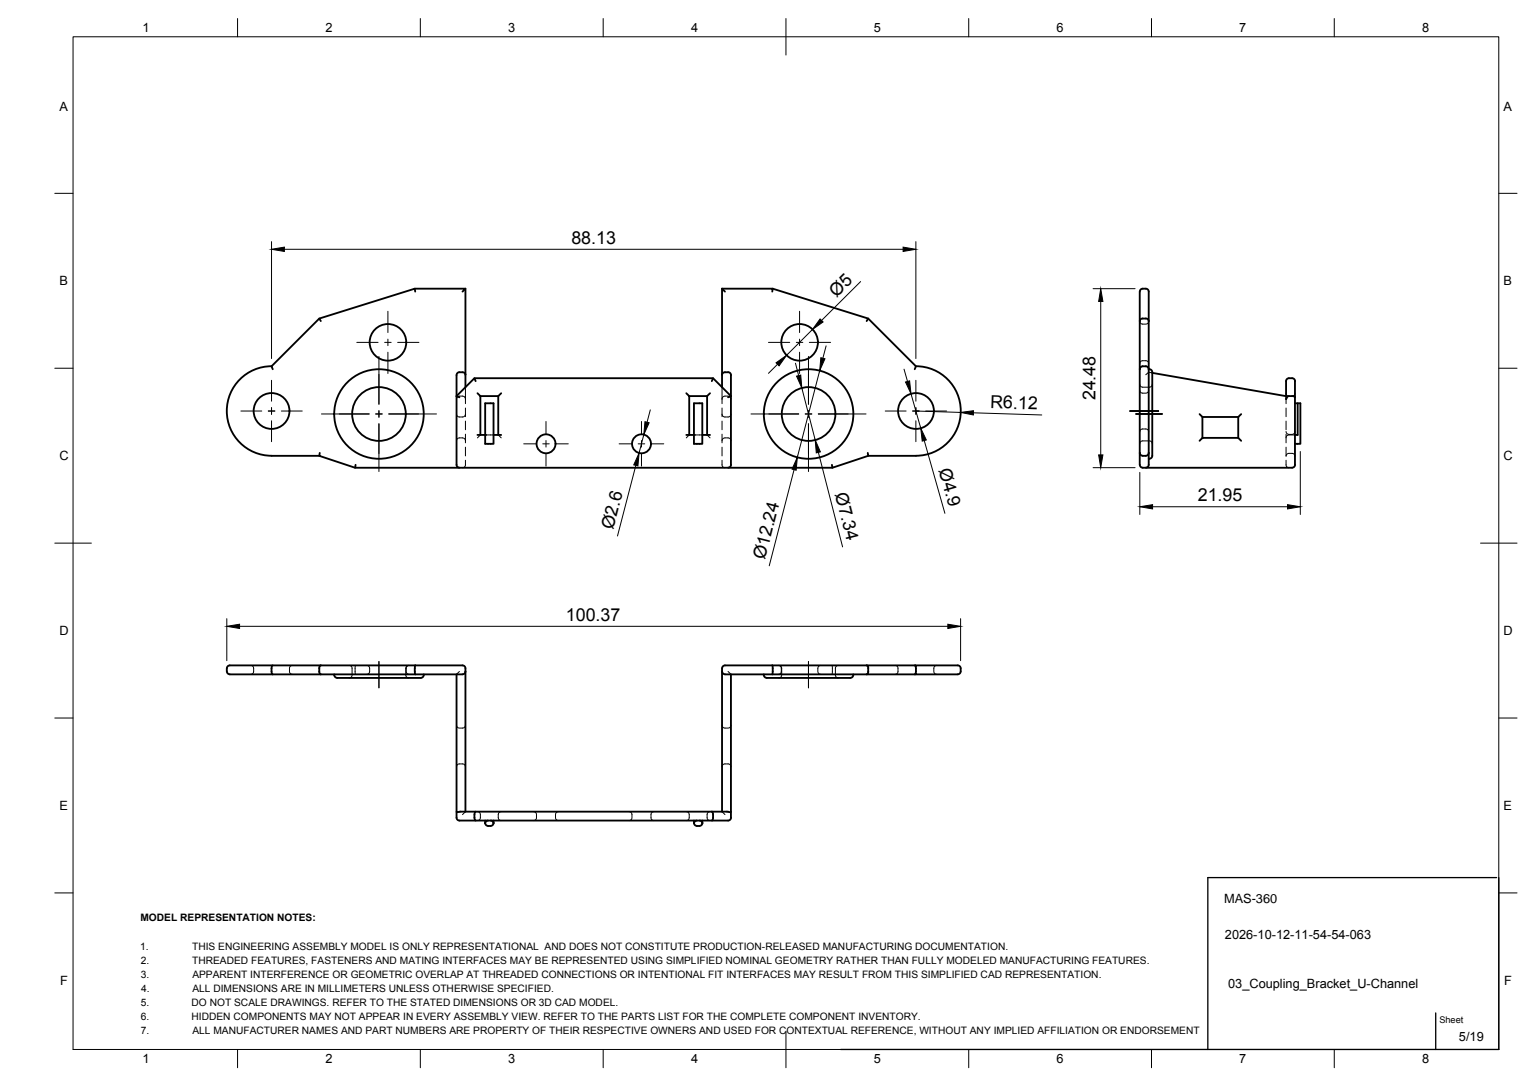
ISO-10303-21;
HEADER;
/* Generated by software containing ST-Developer
 * from STEP Tools, Inc. (www.steptools.com) 
 */

FILE_DESCRIPTION(
/* description */ (''),
/* implementation_level */ '2;1');

FILE_NAME(
/* name */ '03_Coupling_Bracket_U-Channel.step',
/* time_stamp */ '2026-11-04T18:53:29-08:00',
/* author */ (''),
/* organization */ (''),
/* preprocessor_version */ 'ST-DEVELOPER v20.2',
/* originating_system */ 'Autodesk Translation Framework v15.17.0.0',
/* authorisation */ '');

FILE_SCHEMA (('AUTOMOTIVE_DESIGN { 1 0 10303 214 3 1 1 }'));
ENDSEC;

DATA;
#10=MECHANICAL_DESIGN_GEOMETRIC_PRESENTATION_REPRESENTATION('',(#1329),#100031);
#181=SPHERICAL_SURFACE('',#20936,0.4);
#182=SPHERICAL_SURFACE('',#20950,0.4);
#183=SPHERICAL_SURFACE('',#20969,0.4);
#184=SPHERICAL_SURFACE('',#20993,0.4);
#540=CIRCLE('',#20937,0.4);
#541=CIRCLE('',#20938,0.4);
#542=CIRCLE('',#20939,0.399999999999999);
#543=CIRCLE('',#20951,0.400000000000003);
#544=CIRCLE('',#20952,0.399999999999999);
#545=CIRCLE('',#20953,0.400000000000001);
#546=CIRCLE('',#20965,0.4);
#547=CIRCLE('',#20970,0.4);
#548=CIRCLE('',#20971,0.400000000000001);
#549=CIRCLE('',#20972,0.399999999999999);
#550=CIRCLE('',#20977,5.72);
#551=CIRCLE('',#20978,6.12);
#552=CIRCLE('',#20984,6.12);
#553=CIRCLE('',#20992,0.4);
#554=CIRCLE('',#20994,0.399999999999999);
#555=CIRCLE('',#20995,0.4);
#556=CIRCLE('',#21012,0.4);
#557=CIRCLE('',#21014,6.12);
#558=CIRCLE('',#21015,5.72);
#559=CIRCLE('',#21025,6.12);
#560=CIRCLE('',#21032,0.400000000000009);
#561=CIRCLE('',#21033,5.72);
#562=CIRCLE('',#21041,4.072);
#563=CIRCLE('',#21042,2.848);
#564=CIRCLE('',#21043,2.9);
#565=CIRCLE('',#21045,5.72);
#566=CIRCLE('',#21046,0.4);
#567=CIRCLE('',#21047,6.12);
#568=CIRCLE('',#21048,6.12);
#569=CIRCLE('',#21050,4.072);
#570=CIRCLE('',#21052,6.12);
#571=CIRCLE('',#21054,0.4);
#572=CIRCLE('',#21065,5.72);
#573=CIRCLE('',#21067,4.072);
#574=CIRCLE('',#21068,2.9);
#575=CIRCLE('',#21069,2.848);
#576=CIRCLE('',#21071,5.72);
#577=CIRCLE('',#21072,0.4);
#578=CIRCLE('',#21073,6.12);
#579=CIRCLE('',#21074,6.12);
#580=CIRCLE('',#21076,4.072);
#581=CIRCLE('',#21078,6.12);
#582=CIRCLE('',#21080,0.4);
#583=CIRCLE('',#21081,3.672);
#584=CIRCLE('',#21082,3.672);
#585=CIRCLE('',#21084,3.672);
#586=CIRCLE('',#21085,3.672);
#587=CIRCLE('',#21087,0.4);
#588=CIRCLE('',#21089,0.4);
#589=CIRCLE('',#21090,3.672);
#590=CIRCLE('',#21091,3.672);
#591=CIRCLE('',#21093,3.672);
#592=CIRCLE('',#21094,3.672);
#593=CIRCLE('',#21096,0.4);
#594=CIRCLE('',#21098,0.4);
#595=CIRCLE('',#21099,2.448);
#596=CIRCLE('',#21100,2.448);
#597=CIRCLE('',#21102,2.448);
#598=CIRCLE('',#21103,2.448);
#599=CIRCLE('',#21105,2.848);
#600=CIRCLE('',#21106,0.4);
#601=CIRCLE('',#21108,2.9);
#602=CIRCLE('',#21110,0.4);
#603=CIRCLE('',#21111,2.5);
#604=CIRCLE('',#21112,2.5);
#605=CIRCLE('',#21114,2.5);
#606=CIRCLE('',#21115,2.5);
#607=CIRCLE('',#21117,2.9);
#608=CIRCLE('',#21118,0.4);
#609=CIRCLE('',#21120,2.848);
#610=CIRCLE('',#21122,0.4);
#611=CIRCLE('',#21123,2.5);
#612=CIRCLE('',#21124,2.5);
#613=CIRCLE('',#21126,2.5);
#614=CIRCLE('',#21127,2.5);
#615=CIRCLE('',#21129,0.4);
#616=CIRCLE('',#21131,0.4);
#617=CIRCLE('',#21132,2.448);
#618=CIRCLE('',#21133,2.448);
#619=CIRCLE('',#21135,2.448);
#620=CIRCLE('',#21136,2.448);
#621=CIRCLE('',#21138,0.4);
#622=CIRCLE('',#21140,1.7);
#623=CIRCLE('',#21141,0.4);
#624=CIRCLE('',#21142,1.3);
#625=CIRCLE('',#21143,1.3);
#626=CIRCLE('',#21145,1.3);
#627=CIRCLE('',#21146,1.3);
#628=CIRCLE('',#21148,1.7);
#629=CIRCLE('',#21160,1.7);
#630=CIRCLE('',#21161,0.4);
#631=CIRCLE('',#21163,1.7);
#632=CIRCLE('',#21172,0.4);
#633=CIRCLE('',#21173,1.3);
#634=CIRCLE('',#21174,1.3);
#635=CIRCLE('',#21176,1.3);
#636=CIRCLE('',#21177,1.3);
#637=CIRCLE('',#21179,0.4);
#638=CIRCLE('',#21191,0.4);
#639=CIRCLE('',#21196,0.4);
#640=CIRCLE('',#21209,0.4);
#641=CIRCLE('',#21214,0.4);
#642=CIRCLE('',#21217,0.4);
#643=CIRCLE('',#21218,0.4);
#644=CIRCLE('',#21219,0.4);
#645=CIRCLE('',#21221,0.4);
#646=CIRCLE('',#21222,0.4);
#647=CIRCLE('',#21224,0.4);
#648=CIRCLE('',#21225,0.4);
#649=CIRCLE('',#21228,0.4);
#650=CIRCLE('',#21229,0.4);
#651=CIRCLE('',#21231,0.4);
#652=CIRCLE('',#21237,0.4);
#653=CIRCLE('',#21238,0.4);
#654=CIRCLE('',#21239,0.4);
#655=CIRCLE('',#21241,0.4);
#656=CIRCLE('',#21242,0.4);
#657=CIRCLE('',#21244,0.4);
#658=CIRCLE('',#21245,0.4);
#659=CIRCLE('',#21248,0.4);
#660=CIRCLE('',#21249,0.4);
#661=CIRCLE('',#21251,0.4);
#1215=TOROIDAL_SURFACE('',#20976,5.72,0.4);
#1216=TOROIDAL_SURFACE('',#21013,5.72,0.4);
#1217=TOROIDAL_SURFACE('',#21031,5.72,0.4);
#1218=TOROIDAL_SURFACE('',#21044,5.72,0.4);
#1219=TOROIDAL_SURFACE('',#21064,5.72,0.4);
#1220=TOROIDAL_SURFACE('',#21070,5.72,0.4);
#1221=TOROIDAL_SURFACE('',#21079,4.072,0.4);
#1222=TOROIDAL_SURFACE('',#21086,4.072,0.4);
#1223=TOROIDAL_SURFACE('',#21088,4.072,0.4);
#1224=TOROIDAL_SURFACE('',#21095,4.072,0.4);
#1225=TOROIDAL_SURFACE('',#21097,2.848,0.4);
#1226=TOROIDAL_SURFACE('',#21104,2.848,0.4);
#1227=TOROIDAL_SURFACE('',#21109,2.9,0.4);
#1228=TOROIDAL_SURFACE('',#21116,2.9,0.4);
#1229=TOROIDAL_SURFACE('',#21121,2.9,0.4);
#1230=TOROIDAL_SURFACE('',#21128,2.9,0.4);
#1231=TOROIDAL_SURFACE('',#21130,2.848,0.4);
#1232=TOROIDAL_SURFACE('',#21137,2.848,0.4);
#1233=TOROIDAL_SURFACE('',#21139,1.7,0.4);
#1234=TOROIDAL_SURFACE('',#21159,1.7,0.4);
#1235=TOROIDAL_SURFACE('',#21171,1.7,0.4);
#1236=TOROIDAL_SURFACE('',#21178,1.7,0.4);
#1293=SHAPE_REPRESENTATION_RELATIONSHIP('SRR','None',#100103,#1311);
#1311=ADVANCED_BREP_SHAPE_REPRESENTATION('',(#1347),#100015);
#1329=STYLED_ITEM('',(#100201),#1347);
#1347=MANIFOLD_SOLID_BREP('Body1',#20119);
#1399=PLANE('',#20901);
#1400=PLANE('',#20902);
#1401=PLANE('',#20903);
#1402=PLANE('',#20915);
#1403=PLANE('',#20916);
#1404=PLANE('',#20922);
#1405=PLANE('',#20932);
#1406=PLANE('',#20933);
#1407=PLANE('',#20934);
#1408=PLANE('',#20942);
#1409=PLANE('',#20957);
#1410=PLANE('',#20980);
#1411=PLANE('',#20981);
#1412=PLANE('',#20982);
#1413=PLANE('',#20985);
#1414=PLANE('',#20986);
#1415=PLANE('',#21009);
#1416=PLANE('',#21010);
#1417=PLANE('',#21023);
#1418=PLANE('',#21026);
#1419=PLANE('',#21027);
#1420=PLANE('',#21028);
#1421=PLANE('',#21040);
#1422=PLANE('',#21049);
#1423=PLANE('',#21066);
#1424=PLANE('',#21075);
#1425=PLANE('',#21107);
#1426=PLANE('',#21119);
#1427=PLANE('',#21147);
#1428=PLANE('',#21155);
#1429=PLANE('',#21156);
#1430=PLANE('',#21157);
#1431=PLANE('',#21162);
#1432=PLANE('',#21188);
#1433=PLANE('',#21189);
#1434=PLANE('',#21197);
#1435=PLANE('',#21206);
#1436=PLANE('',#21207);
#1437=PLANE('',#21215);
#1438=PLANE('',#21223);
#1439=PLANE('',#21226);
#1440=PLANE('',#21227);
#1441=PLANE('',#21232);
#1442=PLANE('',#21233);
#1443=PLANE('',#21234);
#1444=PLANE('',#21243);
#1445=PLANE('',#21246);
#1446=PLANE('',#21247);
#1447=PLANE('',#21252);
#1448=PLANE('',#21253);
#1449=PLANE('',#21254);
#1450=PLANE('',#21256);
#1451=PLANE('',#21257);
#1452=PLANE('',#21258);
#1453=PLANE('',#21259);
#1454=PLANE('',#21260);
#1717=FACE_BOUND('',#6546,.T.);
#1718=FACE_BOUND('',#6554,.T.);
#1719=FACE_BOUND('',#6565,.T.);
#1720=FACE_BOUND('',#6604,.T.);
#1721=FACE_BOUND('',#6623,.T.);
#1722=FACE_BOUND('',#6624,.T.);
#1723=FACE_BOUND('',#6625,.T.);
#1724=FACE_BOUND('',#6628,.T.);
#1725=FACE_BOUND('',#6638,.T.);
#1726=FACE_BOUND('',#6639,.T.);
#1727=FACE_BOUND('',#6640,.T.);
#1728=FACE_BOUND('',#6643,.T.);
#1729=FACE_BOUND('',#6655,.T.);
#1730=FACE_BOUND('',#6656,.T.);
#1731=FACE_BOUND('',#6657,.T.);
#1732=FACE_BOUND('',#6662,.T.);
#1733=FACE_BOUND('',#6663,.T.);
#1734=FACE_BOUND('',#6664,.T.);
#1735=FACE_BOUND('',#6674,.T.);
#1736=FACE_BOUND('',#6675,.T.);
#1737=FACE_BOUND('',#6676,.T.);
#1738=FACE_BOUND('',#6677,.T.);
#1739=FACE_BOUND('',#6687,.T.);
#1740=FACE_BOUND('',#6688,.T.);
#1741=FACE_BOUND('',#6689,.T.);
#1742=FACE_BOUND('',#6690,.T.);
#1825=ELLIPSE('',#20894,0.565685424949238,0.4);
#1826=ELLIPSE('',#20895,0.565685424949238,0.4);
#1827=ELLIPSE('',#20897,0.565685424949238,0.4);
#1828=ELLIPSE('',#20899,0.565685424949238,0.4);
#1829=ELLIPSE('',#20904,0.565685424949239,0.4);
#1830=ELLIPSE('',#20906,0.406004087997522,0.4);
#1831=ELLIPSE('',#20908,0.565685424949238,0.4);
#1832=ELLIPSE('',#20909,0.565685424949238,0.4);
#1833=ELLIPSE('',#20911,0.565685424949238,0.4);
#1834=ELLIPSE('',#20912,0.565685424949238,0.4);
#1835=ELLIPSE('',#20918,0.522676873082012,0.4);
#1836=ELLIPSE('',#20919,0.406004087997522,0.4);
#1837=ELLIPSE('',#20921,0.406004087997522,0.4);
#1838=ELLIPSE('',#20923,0.574176487625014,0.4);
#1839=ELLIPSE('',#20925,0.565685424949238,0.4);
#1840=ELLIPSE('',#20926,0.565685424949238,0.4);
#1841=ELLIPSE('',#20928,0.565685424949238,0.4);
#1842=ELLIPSE('',#20930,0.565685424949238,0.4);
#1843=ELLIPSE('',#20935,0.565685424949239,0.4);
#1844=ELLIPSE('',#20941,0.565685424949238,0.4);
#1845=ELLIPSE('',#20944,0.405232582893276,0.4);
#1846=ELLIPSE('',#20946,0.565685424949238,0.4);
#1847=ELLIPSE('',#20948,0.56568542494924,0.4);
#1848=ELLIPSE('',#20949,0.405232582893277,0.4);
#1849=ELLIPSE('',#20956,0.405232582893276,0.4);
#1850=ELLIPSE('',#20959,0.565685424949238,0.4);
#1851=ELLIPSE('',#20961,0.404631208637699,0.4);
#1852=ELLIPSE('',#20963,0.41193011418047,0.4);
#1853=ELLIPSE('',#20966,0.405232582893276,0.4);
#1854=ELLIPSE('',#20968,0.405232582893276,0.4);
#1855=ELLIPSE('',#20974,0.565685424949237,0.4);
#1856=ELLIPSE('',#20989,0.43295688011696,0.4);
#1857=ELLIPSE('',#20991,0.565685424949238,0.4);
#1858=ELLIPSE('',#20997,0.405232582893276,0.4);
#1859=ELLIPSE('',#20999,0.522676873082012,0.4);
#1860=ELLIPSE('',#21000,0.406004087997522,0.4);
#1861=ELLIPSE('',#21002,0.565685424949238,0.4);
#1862=ELLIPSE('',#21003,0.565685424949238,0.4);
#1863=ELLIPSE('',#21005,0.565685424949238,0.4);
#1864=ELLIPSE('',#21006,0.565685424949238,0.4);
#1865=ELLIPSE('',#21017,0.41193011418047,0.4);
#1866=ELLIPSE('',#21019,0.404631208637698,0.4);
#1867=ELLIPSE('',#21021,0.56568542494924,0.4);
#1868=ELLIPSE('',#21030,0.405232582893276,0.4);
#1869=ELLIPSE('',#21036,0.411930114180469,0.4);
#1870=ELLIPSE('',#21038,0.404631208637699,0.4);
#1871=ELLIPSE('',#21055,0.405232582893276,0.4);
#1872=ELLIPSE('',#21058,0.565685424949238,0.4);
#1873=ELLIPSE('',#21060,0.404631208637698,0.4);
#1874=ELLIPSE('',#21062,0.411930114180471,0.4);
#1875=ELLIPSE('',#21150,0.574176487625014,0.4);
#1876=ELLIPSE('',#21151,0.432956880116957,0.4);
#1877=ELLIPSE('',#21153,0.432956880116958,0.4);
#1878=ELLIPSE('',#21165,0.432956880116959,0.4);
#1879=ELLIPSE('',#21166,0.432956880116958,0.4);
#1880=ELLIPSE('',#21169,0.432956880116958,0.4);
#1881=ELLIPSE('',#21181,0.565685424949238,0.4);
#1882=ELLIPSE('',#21182,0.565685424949238,0.4);
#1883=ELLIPSE('',#21184,0.565685424949238,0.4);
#1884=ELLIPSE('',#21186,0.565685424949238,0.4);
#1885=ELLIPSE('',#21192,0.565685424949238,0.4);
#1886=ELLIPSE('',#21194,0.565685424949238,0.4);
#1887=ELLIPSE('',#21199,0.565685424949238,0.4);
#1888=ELLIPSE('',#21200,0.565685424949238,0.4);
#1889=ELLIPSE('',#21202,0.565685424949238,0.4);
#1890=ELLIPSE('',#21204,0.565685424949238,0.4);
#1891=ELLIPSE('',#21210,0.565685424949238,0.4);
#1892=ELLIPSE('',#21212,0.565685424949238,0.4);
#2284=LINE('',#60104,#3571);
#2285=LINE('',#60108,#3572);
#2286=LINE('',#60112,#3573);
#2287=LINE('',#60114,#3574);
#2288=LINE('',#60118,#3575);
#2289=LINE('',#60120,#3576);
#2290=LINE('',#60123,#3577);
#2291=LINE('',#60124,#3578);
#2292=LINE('',#60127,#3579);
#2293=LINE('',#60129,#3580);
#2294=LINE('',#60130,#3581);
#2295=LINE('',#60133,#3582);
#2296=LINE('',#60134,#3583);
#2297=LINE('',#60138,#3584);
#2298=LINE('',#60142,#3585);
#2299=LINE('',#60144,#3586);
#2300=LINE('',#60146,#3587);
#2301=LINE('',#60147,#3588);
#2302=LINE('',#60168,#3589);
#2303=LINE('',#60172,#3590);
#2304=LINE('',#60175,#3591);
#2305=LINE('',#60180,#3592);
#2306=LINE('',#60184,#3593);
#2307=LINE('',#60186,#3594);
#2308=LINE('',#60187,#3595);
#2309=LINE('',#60189,#3596);
#2310=LINE('',#60193,#3597);
#2311=LINE('',#60195,#3598);
#2312=LINE('',#60197,#3599);
#2313=LINE('',#60199,#3600);
#2314=LINE('',#60201,#3601);
#2315=LINE('',#60202,#3602);
#2316=LINE('',#60208,#3603);
#2317=LINE('',#60229,#3604);
#2318=LINE('',#60232,#3605);
#2319=LINE('',#60237,#3606);
#2320=LINE('',#60239,#3607);
#2321=LINE('',#60240,#3608);
#2322=LINE('',#60244,#3609);
#2323=LINE('',#60248,#3610);
#2324=LINE('',#60252,#3611);
#2325=LINE('',#60254,#3612);
#2326=LINE('',#60258,#3613);
#2327=LINE('',#60260,#3614);
#2328=LINE('',#60263,#3615);
#2329=LINE('',#60264,#3616);
#2330=LINE('',#60267,#3617);
#2331=LINE('',#60269,#3618);
#2332=LINE('',#60270,#3619);
#2333=LINE('',#60273,#3620);
#2334=LINE('',#60274,#3621);
#2335=LINE('',#60277,#3622);
#2336=LINE('',#60279,#3623);
#2337=LINE('',#60281,#3624);
#2338=LINE('',#60283,#3625);
#2339=LINE('',#60294,#3626);
#2340=LINE('',#60297,#3627);
#2341=LINE('',#60299,#3628);
#2342=LINE('',#60301,#3629);
#2343=LINE('',#60303,#3630);
#2344=LINE('',#60305,#3631);
#2345=LINE('',#60307,#3632);
#2346=LINE('',#60309,#3633);
#2347=LINE('',#60311,#3634);
#2348=LINE('',#60313,#3635);
#2349=LINE('',#60315,#3636);
#2350=LINE('',#60316,#3637);
#2351=LINE('',#60319,#3638);
#2352=LINE('',#60324,#3639);
#2353=LINE('',#60328,#3640);
#2354=LINE('',#60338,#3641);
#2355=LINE('',#60341,#3642);
#2356=LINE('',#60344,#3643);
#2357=LINE('',#60345,#3644);
#2358=LINE('',#60348,#3645);
#2359=LINE('',#60352,#3646);
#2360=LINE('',#60355,#3647);
#2361=LINE('',#60358,#3648);
#2362=LINE('',#60361,#3649);
#2363=LINE('',#60365,#3650);
#2364=LINE('',#60369,#3651);
#2365=LINE('',#60373,#3652);
#2366=LINE('',#60375,#3653);
#2367=LINE('',#60384,#3654);
#2368=LINE('',#60419,#3655);
#2369=LINE('',#60420,#3656);
#2370=LINE('',#60423,#3657);
#2371=LINE('',#60424,#3658);
#2372=LINE('',#60427,#3659);
#2373=LINE('',#60428,#3660);
#2374=LINE('',#60431,#3661);
#2375=LINE('',#60432,#3662);
#2376=LINE('',#60435,#3663);
#2377=LINE('',#60439,#3664);
#2378=LINE('',#60440,#3665);
#2379=LINE('',#60442,#3666);
#2380=LINE('',#60444,#3667);
#2381=LINE('',#60448,#3668);
#2382=LINE('',#60454,#3669);
#2383=LINE('',#60462,#3670);
#2384=LINE('',#60468,#3671);
#2385=LINE('',#60472,#3672);
#2386=LINE('',#60475,#3673);
#2387=LINE('',#60480,#3674);
#2388=LINE('',#60484,#3675);
#2389=LINE('',#60486,#3676);
#2390=LINE('',#60487,#3677);
#2391=LINE('',#60489,#3678);
#2392=LINE('',#60492,#3679);
#2393=LINE('',#60494,#3680);
#2394=LINE('',#60495,#3681);
#2395=LINE('',#60496,#3682);
#2396=LINE('',#60501,#3683);
#2397=LINE('',#60502,#3684);
#2398=LINE('',#60538,#3685);
#2399=LINE('',#60541,#3686);
#2400=LINE('',#60544,#3687);
#2401=LINE('',#60547,#3688);
#2402=LINE('',#60550,#3689);
#2403=LINE('',#60553,#3690);
#2404=LINE('',#60554,#3691);
#2405=LINE('',#60557,#3692);
#2406=LINE('',#60558,#3693);
#2407=LINE('',#60561,#3694);
#2408=LINE('',#60565,#3695);
#2409=LINE('',#60566,#3696);
#2410=LINE('',#60569,#3697);
#2411=LINE('',#60570,#3698);
#2412=LINE('',#60572,#3699);
#2413=LINE('',#60575,#3700);
#2414=LINE('',#60611,#3701);
#2415=LINE('',#60614,#3702);
#2416=LINE('',#60618,#3703);
#2417=LINE('',#60621,#3704);
#2418=LINE('',#60642,#3705);
#2419=LINE('',#60648,#3706);
#2420=LINE('',#60651,#3707);
#2421=LINE('',#60654,#3708);
#2422=LINE('',#60658,#3709);
#2423=LINE('',#60662,#3710);
#2424=LINE('',#60666,#3711);
#2425=LINE('',#60717,#3712);
#2426=LINE('',#60727,#3713);
#2427=LINE('',#60741,#3714);
#2428=LINE('',#60758,#3715);
#2429=LINE('',#60777,#3716);
#2430=LINE('',#60783,#3717);
#2431=LINE('',#60797,#3718);
#2432=LINE('',#60811,#3719);
#2433=LINE('',#60827,#3720);
#2434=LINE('',#60831,#3721);
#2435=LINE('',#60832,#3722);
#2436=LINE('',#60833,#3723);
#2437=LINE('',#60835,#3724);
#2438=LINE('',#60836,#3725);
#2439=LINE('',#60841,#3726);
#2440=LINE('',#60843,#3727);
#2441=LINE('',#60845,#3728);
#2442=LINE('',#60846,#3729);
#2443=LINE('',#60849,#3730);
#2444=LINE('',#60851,#3731);
#2445=LINE('',#60853,#3732);
#2446=LINE('',#60854,#3733);
#2447=LINE('',#60857,#3734);
#2448=LINE('',#60863,#3735);
#2449=LINE('',#60865,#3736);
#2450=LINE('',#60868,#3737);
#2451=LINE('',#60869,#3738);
#2452=LINE('',#60872,#3739);
#2453=LINE('',#60873,#3740);
#2454=LINE('',#60875,#3741);
#2455=LINE('',#60883,#3742);
#2456=LINE('',#60885,#3743);
#2457=LINE('',#60887,#3744);
#2458=LINE('',#60888,#3745);
#2459=LINE('',#60891,#3746);
#2460=LINE('',#60893,#3747);
#2461=LINE('',#60895,#3748);
#2462=LINE('',#60897,#3749);
#2463=LINE('',#60899,#3750);
#2464=LINE('',#60901,#3751);
#2465=LINE('',#60903,#3752);
#2466=LINE('',#60904,#3753);
#2467=LINE('',#60907,#3754);
#2468=LINE('',#60909,#3755);
#2469=LINE('',#60911,#3756);
#2470=LINE('',#60913,#3757);
#2471=LINE('',#60915,#3758);
#2472=LINE('',#60917,#3759);
#2473=LINE('',#60919,#3760);
#2474=LINE('',#60920,#3761);
#2475=LINE('',#60938,#3762);
#2476=LINE('',#60948,#3763);
#2477=LINE('',#60952,#3764);
#2478=LINE('',#60956,#3765);
#2479=LINE('',#60959,#3766);
#2480=LINE('',#60962,#3767);
#2481=LINE('',#60964,#3768);
#2482=LINE('',#60965,#3769);
#2483=LINE('',#60968,#3770);
#2484=LINE('',#60969,#3771);
#2485=LINE('',#60978,#3772);
#2486=LINE('',#60980,#3773);
#2487=LINE('',#60985,#3774);
#2488=LINE('',#60989,#3775);
#2489=LINE('',#60993,#3776);
#2490=LINE('',#60996,#3777);
#2491=LINE('',#60999,#3778);
#2492=LINE('',#61001,#3779);
#2493=LINE('',#61002,#3780);
#2494=LINE('',#61005,#3781);
#2495=LINE('',#61006,#3782);
#2496=LINE('',#61015,#3783);
#2497=LINE('',#61017,#3784);
#2498=LINE('',#61023,#3785);
#2499=LINE('',#61027,#3786);
#2500=LINE('',#61030,#3787);
#2501=LINE('',#61035,#3788);
#2502=LINE('',#61039,#3789);
#2503=LINE('',#61044,#3790);
#2504=LINE('',#61045,#3791);
#2505=LINE('',#61047,#3792);
#2506=LINE('',#61050,#3793);
#2507=LINE('',#61055,#3794);
#2508=LINE('',#61060,#3795);
#2509=LINE('',#61061,#3796);
#2510=LINE('',#61062,#3797);
#2511=LINE('',#61064,#3798);
#2512=LINE('',#61066,#3799);
#2513=LINE('',#61069,#3800);
#2514=LINE('',#61075,#3801);
#2515=LINE('',#61079,#3802);
#2516=LINE('',#61082,#3803);
#2517=LINE('',#61087,#3804);
#2518=LINE('',#61091,#3805);
#2519=LINE('',#61096,#3806);
#2520=LINE('',#61097,#3807);
#2521=LINE('',#61099,#3808);
#2522=LINE('',#61102,#3809);
#2523=LINE('',#61107,#3810);
#2524=LINE('',#61112,#3811);
#2525=LINE('',#61113,#3812);
#2526=LINE('',#61114,#3813);
#2527=LINE('',#61116,#3814);
#2528=LINE('',#61118,#3815);
#2529=LINE('',#61121,#3816);
#3571=VECTOR('',#23949,10.);
#3572=VECTOR('',#23952,10.);
#3573=VECTOR('',#23957,10.);
#3574=VECTOR('',#23958,10.);
#3575=VECTOR('',#23963,10.);
#3576=VECTOR('',#23964,10.);
#3577=VECTOR('',#23969,10.);
#3578=VECTOR('',#23970,10.);
#3579=VECTOR('',#23973,10.);
#3580=VECTOR('',#23974,10.);
#3581=VECTOR('',#23975,10.);
#3582=VECTOR('',#23978,10.);
#3583=VECTOR('',#23979,10.);
#3584=VECTOR('',#23982,10.);
#3585=VECTOR('',#23985,10.);
#3586=VECTOR('',#23986,10.);
#3587=VECTOR('',#23987,10.);
#3588=VECTOR('',#23988,10.);
#3589=VECTOR('',#23993,10.);
#3590=VECTOR('',#23996,10.);
#3591=VECTOR('',#23999,10.);
#3592=VECTOR('',#24004,10.);
#3593=VECTOR('',#24011,10.);
#3594=VECTOR('',#24014,10.);
#3595=VECTOR('',#24015,10.);
#3596=VECTOR('',#24018,10.);
#3597=VECTOR('',#24021,10.);
#3598=VECTOR('',#24022,10.);
#3599=VECTOR('',#24023,10.);
#3600=VECTOR('',#24024,10.);
#3601=VECTOR('',#24025,10.);
#3602=VECTOR('',#24026,10.);
#3603=VECTOR('',#24033,10.);
#3604=VECTOR('',#24036,10.);
#3605=VECTOR('',#24039,10.);
#3606=VECTOR('',#24044,10.);
#3607=VECTOR('',#24045,10.);
#3608=VECTOR('',#24046,10.);
#3609=VECTOR('',#24049,10.);
#3610=VECTOR('',#24052,10.);
#3611=VECTOR('',#24057,10.);
#3612=VECTOR('',#24058,10.);
#3613=VECTOR('',#24063,10.);
#3614=VECTOR('',#24064,10.);
#3615=VECTOR('',#24069,10.);
#3616=VECTOR('',#24070,10.);
#3617=VECTOR('',#24073,10.);
#3618=VECTOR('',#24074,10.);
#3619=VECTOR('',#24075,10.);
#3620=VECTOR('',#24078,10.);
#3621=VECTOR('',#24079,10.);
#3622=VECTOR('',#24082,10.);
#3623=VECTOR('',#24083,10.);
#3624=VECTOR('',#24084,10.);
#3625=VECTOR('',#24085,10.);
#3626=VECTOR('',#24100,10.);
#3627=VECTOR('',#24103,10.);
#3628=VECTOR('',#24104,10.);
#3629=VECTOR('',#24105,10.);
#3630=VECTOR('',#24106,10.);
#3631=VECTOR('',#24107,10.);
#3632=VECTOR('',#24108,10.);
#3633=VECTOR('',#24109,10.);
#3634=VECTOR('',#24110,10.);
#3635=VECTOR('',#24111,10.);
#3636=VECTOR('',#24112,10.);
#3637=VECTOR('',#24113,10.);
#3638=VECTOR('',#24116,10.);
#3639=VECTOR('',#24123,10.);
#3640=VECTOR('',#24128,10.);
#3641=VECTOR('',#24143,10.);
#3642=VECTOR('',#24146,10.);
#3643=VECTOR('',#24149,10.);
#3644=VECTOR('',#24150,10.);
#3645=VECTOR('',#24153,10.);
#3646=VECTOR('',#24158,10.);
#3647=VECTOR('',#24161,10.);
#3648=VECTOR('',#24164,10.);
#3649=VECTOR('',#24167,10.);
#3650=VECTOR('',#24170,10.);
#3651=VECTOR('',#24173,10.);
#3652=VECTOR('',#24178,10.);
#3653=VECTOR('',#24181,10.);
#3654=VECTOR('',#24196,10.);
#3655=VECTOR('',#24205,10.);
#3656=VECTOR('',#24206,10.);
#3657=VECTOR('',#24209,10.);
#3658=VECTOR('',#24210,10.);
#3659=VECTOR('',#24213,10.);
#3660=VECTOR('',#24214,10.);
#3661=VECTOR('',#24217,10.);
#3662=VECTOR('',#24218,10.);
#3663=VECTOR('',#24221,10.);
#3664=VECTOR('',#24226,10.);
#3665=VECTOR('',#24227,10.);
#3666=VECTOR('',#24230,10.);
#3667=VECTOR('',#24233,10.);
#3668=VECTOR('',#24238,10.);
#3669=VECTOR('',#24245,10.);
#3670=VECTOR('',#24256,10.);
#3671=VECTOR('',#24263,10.);
#3672=VECTOR('',#24266,10.);
#3673=VECTOR('',#24269,10.);
#3674=VECTOR('',#24274,10.);
#3675=VECTOR('',#24281,10.);
#3676=VECTOR('',#24284,10.);
#3677=VECTOR('',#24285,10.);
#3678=VECTOR('',#24288,10.);
#3679=VECTOR('',#24291,10.);
#3680=VECTOR('',#24292,10.);
#3681=VECTOR('',#24293,10.);
#3682=VECTOR('',#24294,10.);
#3683=VECTOR('',#24299,10.);
#3684=VECTOR('',#24300,10.);
#3685=VECTOR('',#24309,10.);
#3686=VECTOR('',#24312,10.);
#3687=VECTOR('',#24315,10.);
#3688=VECTOR('',#24318,10.);
#3689=VECTOR('',#24321,10.);
#3690=VECTOR('',#24326,10.);
#3691=VECTOR('',#24327,10.);
#3692=VECTOR('',#24330,10.);
#3693=VECTOR('',#24331,10.);
#3694=VECTOR('',#24334,10.);
#3695=VECTOR('',#24339,10.);
#3696=VECTOR('',#24340,10.);
#3697=VECTOR('',#24343,10.);
#3698=VECTOR('',#24344,10.);
#3699=VECTOR('',#24347,10.);
#3700=VECTOR('',#24350,10.);
#3701=VECTOR('',#24361,10.);
#3702=VECTOR('',#24364,10.);
#3703=VECTOR('',#24369,10.);
#3704=VECTOR('',#24374,10.);
#3705=VECTOR('',#24399,6.12);
#3706=VECTOR('',#24406,10.);
#3707=VECTOR('',#24411,10.);
#3708=VECTOR('',#24414,10.);
#3709=VECTOR('',#24419,10.);
#3710=VECTOR('',#24424,10.);
#3711=VECTOR('',#24429,10.);
#3712=VECTOR('',#24458,6.12);
#3713=VECTOR('',#24471,3.672);
#3714=VECTOR('',#24490,3.672);
#3715=VECTOR('',#24513,2.448);
#3716=VECTOR('',#24538,2.5);
#3717=VECTOR('',#24547,10.);
#3718=VECTOR('',#24564,2.5);
#3719=VECTOR('',#24583,2.448);
#3720=VECTOR('',#24604,1.3);
#3721=VECTOR('',#24607,10.);
#3722=VECTOR('',#24608,10.);
#3723=VECTOR('',#24609,10.);
#3724=VECTOR('',#24610,10.);
#3725=VECTOR('',#24611,10.);
#3726=VECTOR('',#24614,10.);
#3727=VECTOR('',#24615,10.);
#3728=VECTOR('',#24616,10.);
#3729=VECTOR('',#24617,10.);
#3730=VECTOR('',#24618,10.);
#3731=VECTOR('',#24619,10.);
#3732=VECTOR('',#24620,10.);
#3733=VECTOR('',#24621,10.);
#3734=VECTOR('',#24624,10.);
#3735=VECTOR('',#24633,10.);
#3736=VECTOR('',#24636,10.);
#3737=VECTOR('',#24639,10.);
#3738=VECTOR('',#24640,10.);
#3739=VECTOR('',#24643,10.);
#3740=VECTOR('',#24644,10.);
#3741=VECTOR('',#24647,10.);
#3742=VECTOR('',#24658,10.);
#3743=VECTOR('',#24659,10.);
#3744=VECTOR('',#24660,10.);
#3745=VECTOR('',#24661,10.);
#3746=VECTOR('',#24662,10.);
#3747=VECTOR('',#24663,10.);
#3748=VECTOR('',#24664,10.);
#3749=VECTOR('',#24665,10.);
#3750=VECTOR('',#24666,10.);
#3751=VECTOR('',#24667,10.);
#3752=VECTOR('',#24668,10.);
#3753=VECTOR('',#24669,10.);
#3754=VECTOR('',#24670,10.);
#3755=VECTOR('',#24671,10.);
#3756=VECTOR('',#24672,10.);
#3757=VECTOR('',#24673,10.);
#3758=VECTOR('',#24674,10.);
#3759=VECTOR('',#24675,10.);
#3760=VECTOR('',#24676,10.);
#3761=VECTOR('',#24677,10.);
#3762=VECTOR('',#24704,1.3);
#3763=VECTOR('',#24717,10.);
#3764=VECTOR('',#24722,10.);
#3765=VECTOR('',#24727,10.);
#3766=VECTOR('',#24732,10.);
#3767=VECTOR('',#24735,10.);
#3768=VECTOR('',#24736,10.);
#3769=VECTOR('',#24737,10.);
#3770=VECTOR('',#24740,10.);
#3771=VECTOR('',#24741,10.);
#3772=VECTOR('',#24756,10.);
#3773=VECTOR('',#24759,10.);
#3774=VECTOR('',#24764,10.);
#3775=VECTOR('',#24769,10.);
#3776=VECTOR('',#24774,10.);
#3777=VECTOR('',#24779,10.);
#3778=VECTOR('',#24782,10.);
#3779=VECTOR('',#24783,10.);
#3780=VECTOR('',#24784,10.);
#3781=VECTOR('',#24787,10.);
#3782=VECTOR('',#24788,10.);
#3783=VECTOR('',#24803,10.);
#3784=VECTOR('',#24806,10.);
#3785=VECTOR('',#24811,10.);
#3786=VECTOR('',#24814,10.);
#3787=VECTOR('',#24817,10.);
#3788=VECTOR('',#24822,10.);
#3789=VECTOR('',#24827,10.);
#3790=VECTOR('',#24832,10.);
#3791=VECTOR('',#24833,10.);
#3792=VECTOR('',#24836,10.);
#3793=VECTOR('',#24839,10.);
#3794=VECTOR('',#24844,10.);
#3795=VECTOR('',#24849,10.);
#3796=VECTOR('',#24850,10.);
#3797=VECTOR('',#24851,10.);
#3798=VECTOR('',#24854,10.);
#3799=VECTOR('',#24857,10.);
#3800=VECTOR('',#24862,10.);
#3801=VECTOR('',#24867,10.);
#3802=VECTOR('',#24870,10.);
#3803=VECTOR('',#24873,10.);
#3804=VECTOR('',#24878,10.);
#3805=VECTOR('',#24883,10.);
#3806=VECTOR('',#24888,10.);
#3807=VECTOR('',#24889,10.);
#3808=VECTOR('',#24892,10.);
#3809=VECTOR('',#24895,10.);
#3810=VECTOR('',#24900,10.);
#3811=VECTOR('',#24905,10.);
#3812=VECTOR('',#24906,10.);
#3813=VECTOR('',#24907,10.);
#3814=VECTOR('',#24910,10.);
#3815=VECTOR('',#24913,10.);
#3816=VECTOR('',#24918,10.);
#4671=CYLINDRICAL_SURFACE('',#20893,0.4);
#4672=CYLINDRICAL_SURFACE('',#20896,0.4);
#4673=CYLINDRICAL_SURFACE('',#20898,0.4);
#4674=CYLINDRICAL_SURFACE('',#20900,0.4);
#4675=CYLINDRICAL_SURFACE('',#20905,0.4);
#4676=CYLINDRICAL_SURFACE('',#20907,0.4);
#4677=CYLINDRICAL_SURFACE('',#20910,0.4);
#4678=CYLINDRICAL_SURFACE('',#20913,0.4);
#4679=CYLINDRICAL_SURFACE('',#20914,0.4);
#4680=CYLINDRICAL_SURFACE('',#20917,0.4);
#4681=CYLINDRICAL_SURFACE('',#20920,0.4);
#4682=CYLINDRICAL_SURFACE('',#20924,0.4);
#4683=CYLINDRICAL_SURFACE('',#20927,0.4);
#4684=CYLINDRICAL_SURFACE('',#20929,0.4);
#4685=CYLINDRICAL_SURFACE('',#20931,0.4);
#4686=CYLINDRICAL_SURFACE('',#20940,0.4);
#4687=CYLINDRICAL_SURFACE('',#20943,0.4);
#4688=CYLINDRICAL_SURFACE('',#20945,0.4);
#4689=CYLINDRICAL_SURFACE('',#20947,0.4);
#4690=CYLINDRICAL_SURFACE('',#20954,0.4);
#4691=CYLINDRICAL_SURFACE('',#20955,0.4);
#4692=CYLINDRICAL_SURFACE('',#20958,0.4);
#4693=CYLINDRICAL_SURFACE('',#20960,0.4);
#4694=CYLINDRICAL_SURFACE('',#20962,0.4);
#4695=CYLINDRICAL_SURFACE('',#20964,0.4);
#4696=CYLINDRICAL_SURFACE('',#20967,0.4);
#4697=CYLINDRICAL_SURFACE('',#20973,0.4);
#4698=CYLINDRICAL_SURFACE('',#20975,0.4);
#4699=CYLINDRICAL_SURFACE('',#20979,0.4);
#4700=CYLINDRICAL_SURFACE('',#20983,6.12);
#4701=CYLINDRICAL_SURFACE('',#20987,0.4);
#4702=CYLINDRICAL_SURFACE('',#20988,0.4);
#4703=CYLINDRICAL_SURFACE('',#20990,0.4);
#4704=CYLINDRICAL_SURFACE('',#20996,0.4);
#4705=CYLINDRICAL_SURFACE('',#20998,0.4);
#4706=CYLINDRICAL_SURFACE('',#21001,0.4);
#4707=CYLINDRICAL_SURFACE('',#21004,0.4);
#4708=CYLINDRICAL_SURFACE('',#21007,0.4);
#4709=CYLINDRICAL_SURFACE('',#21008,0.4);
#4710=CYLINDRICAL_SURFACE('',#21011,0.4);
#4711=CYLINDRICAL_SURFACE('',#21016,0.4);
#4712=CYLINDRICAL_SURFACE('',#21018,0.4);
#4713=CYLINDRICAL_SURFACE('',#21020,0.4);
#4714=CYLINDRICAL_SURFACE('',#21022,0.4);
#4715=CYLINDRICAL_SURFACE('',#21024,6.12);
#4716=CYLINDRICAL_SURFACE('',#21029,0.4);
#4717=CYLINDRICAL_SURFACE('',#21034,0.4);
#4718=CYLINDRICAL_SURFACE('',#21035,0.4);
#4719=CYLINDRICAL_SURFACE('',#21037,0.4);
#4720=CYLINDRICAL_SURFACE('',#21039,0.4);
#4721=CYLINDRICAL_SURFACE('',#21051,6.12);
#4722=CYLINDRICAL_SURFACE('',#21053,0.4);
#4723=CYLINDRICAL_SURFACE('',#21056,0.4);
#4724=CYLINDRICAL_SURFACE('',#21057,0.4);
#4725=CYLINDRICAL_SURFACE('',#21059,0.4);
#4726=CYLINDRICAL_SURFACE('',#21061,0.4);
#4727=CYLINDRICAL_SURFACE('',#21063,0.4);
#4728=CYLINDRICAL_SURFACE('',#21077,6.12);
#4729=CYLINDRICAL_SURFACE('',#21083,3.672);
#4730=CYLINDRICAL_SURFACE('',#21092,3.672);
#4731=CYLINDRICAL_SURFACE('',#21101,2.448);
#4732=CYLINDRICAL_SURFACE('',#21113,2.5);
#4733=CYLINDRICAL_SURFACE('',#21125,2.5);
#4734=CYLINDRICAL_SURFACE('',#21134,2.448);
#4735=CYLINDRICAL_SURFACE('',#21144,1.3);
#4736=CYLINDRICAL_SURFACE('',#21149,0.4);
#4737=CYLINDRICAL_SURFACE('',#21152,0.4);
#4738=CYLINDRICAL_SURFACE('',#21154,0.4);
#4739=CYLINDRICAL_SURFACE('',#21158,0.4);
#4740=CYLINDRICAL_SURFACE('',#21164,0.4);
#4741=CYLINDRICAL_SURFACE('',#21167,0.4);
#4742=CYLINDRICAL_SURFACE('',#21168,0.4);
#4743=CYLINDRICAL_SURFACE('',#21170,0.4);
#4744=CYLINDRICAL_SURFACE('',#21175,1.3);
#4745=CYLINDRICAL_SURFACE('',#21180,0.4);
#4746=CYLINDRICAL_SURFACE('',#21183,0.4);
#4747=CYLINDRICAL_SURFACE('',#21185,0.4);
#4748=CYLINDRICAL_SURFACE('',#21187,0.4);
#4749=CYLINDRICAL_SURFACE('',#21190,0.4);
#4750=CYLINDRICAL_SURFACE('',#21193,0.4);
#4751=CYLINDRICAL_SURFACE('',#21195,0.4);
#4752=CYLINDRICAL_SURFACE('',#21198,0.4);
#4753=CYLINDRICAL_SURFACE('',#21201,0.4);
#4754=CYLINDRICAL_SURFACE('',#21203,0.4);
#4755=CYLINDRICAL_SURFACE('',#21205,0.4);
#4756=CYLINDRICAL_SURFACE('',#21208,0.4);
#4757=CYLINDRICAL_SURFACE('',#21211,0.4);
#4758=CYLINDRICAL_SURFACE('',#21213,0.4);
#4759=CYLINDRICAL_SURFACE('',#21216,0.4);
#4760=CYLINDRICAL_SURFACE('',#21220,0.4);
#4761=CYLINDRICAL_SURFACE('',#21230,0.4);
#4762=CYLINDRICAL_SURFACE('',#21235,0.4);
#4763=CYLINDRICAL_SURFACE('',#21236,0.4);
#4764=CYLINDRICAL_SURFACE('',#21240,0.4);
#4765=CYLINDRICAL_SURFACE('',#21250,0.4);
#4766=CYLINDRICAL_SURFACE('',#21255,0.4);
#5359=FACE_OUTER_BOUND('',#6539,.T.);
#5360=FACE_OUTER_BOUND('',#6540,.T.);
#5361=FACE_OUTER_BOUND('',#6541,.T.);
#5362=FACE_OUTER_BOUND('',#6542,.T.);
#5363=FACE_OUTER_BOUND('',#6543,.T.);
#5364=FACE_OUTER_BOUND('',#6544,.T.);
#5365=FACE_OUTER_BOUND('',#6545,.T.);
#5366=FACE_OUTER_BOUND('',#6547,.T.);
#5367=FACE_OUTER_BOUND('',#6548,.T.);
#5368=FACE_OUTER_BOUND('',#6549,.T.);
#5369=FACE_OUTER_BOUND('',#6550,.T.);
#5370=FACE_OUTER_BOUND('',#6551,.T.);
#5371=FACE_OUTER_BOUND('',#6552,.T.);
#5372=FACE_OUTER_BOUND('',#6553,.T.);
#5373=FACE_OUTER_BOUND('',#6555,.T.);
#5374=FACE_OUTER_BOUND('',#6556,.T.);
#5375=FACE_OUTER_BOUND('',#6557,.T.);
#5376=FACE_OUTER_BOUND('',#6558,.T.);
#5377=FACE_OUTER_BOUND('',#6559,.T.);
#5378=FACE_OUTER_BOUND('',#6560,.T.);
#5379=FACE_OUTER_BOUND('',#6561,.T.);
#5380=FACE_OUTER_BOUND('',#6562,.T.);
#5381=FACE_OUTER_BOUND('',#6563,.T.);
#5382=FACE_OUTER_BOUND('',#6564,.T.);
#5383=FACE_OUTER_BOUND('',#6566,.T.);
#5384=FACE_OUTER_BOUND('',#6567,.T.);
#5385=FACE_OUTER_BOUND('',#6568,.T.);
#5386=FACE_OUTER_BOUND('',#6569,.T.);
#5387=FACE_OUTER_BOUND('',#6570,.T.);
#5388=FACE_OUTER_BOUND('',#6571,.T.);
#5389=FACE_OUTER_BOUND('',#6572,.T.);
#5390=FACE_OUTER_BOUND('',#6573,.T.);
#5391=FACE_OUTER_BOUND('',#6574,.T.);
#5392=FACE_OUTER_BOUND('',#6575,.T.);
#5393=FACE_OUTER_BOUND('',#6576,.T.);
#5394=FACE_OUTER_BOUND('',#6577,.T.);
#5395=FACE_OUTER_BOUND('',#6578,.T.);
#5396=FACE_OUTER_BOUND('',#6579,.T.);
#5397=FACE_OUTER_BOUND('',#6580,.T.);
#5398=FACE_OUTER_BOUND('',#6581,.T.);
#5399=FACE_OUTER_BOUND('',#6582,.T.);
#5400=FACE_OUTER_BOUND('',#6583,.T.);
#5401=FACE_OUTER_BOUND('',#6584,.T.);
#5402=FACE_OUTER_BOUND('',#6585,.T.);
#5403=FACE_OUTER_BOUND('',#6586,.T.);
#5404=FACE_OUTER_BOUND('',#6587,.T.);
#5405=FACE_OUTER_BOUND('',#6588,.T.);
#5406=FACE_OUTER_BOUND('',#6589,.T.);
#5407=FACE_OUTER_BOUND('',#6590,.T.);
#5408=FACE_OUTER_BOUND('',#6591,.T.);
#5409=FACE_OUTER_BOUND('',#6592,.T.);
#5410=FACE_OUTER_BOUND('',#6593,.T.);
#5411=FACE_OUTER_BOUND('',#6594,.T.);
#5412=FACE_OUTER_BOUND('',#6595,.T.);
#5413=FACE_OUTER_BOUND('',#6596,.T.);
#5414=FACE_OUTER_BOUND('',#6597,.T.);
#5415=FACE_OUTER_BOUND('',#6598,.T.);
#5416=FACE_OUTER_BOUND('',#6599,.T.);
#5417=FACE_OUTER_BOUND('',#6600,.T.);
#5418=FACE_OUTER_BOUND('',#6601,.T.);
#5419=FACE_OUTER_BOUND('',#6602,.T.);
#5420=FACE_OUTER_BOUND('',#6603,.T.);
#5421=FACE_OUTER_BOUND('',#6605,.T.);
#5422=FACE_OUTER_BOUND('',#6606,.T.);
#5423=FACE_OUTER_BOUND('',#6607,.T.);
#5424=FACE_OUTER_BOUND('',#6608,.T.);
#5425=FACE_OUTER_BOUND('',#6609,.T.);
#5426=FACE_OUTER_BOUND('',#6610,.T.);
#5427=FACE_OUTER_BOUND('',#6611,.T.);
#5428=FACE_OUTER_BOUND('',#6612,.T.);
#5429=FACE_OUTER_BOUND('',#6613,.T.);
#5430=FACE_OUTER_BOUND('',#6614,.T.);
#5431=FACE_OUTER_BOUND('',#6615,.T.);
#5432=FACE_OUTER_BOUND('',#6616,.T.);
#5433=FACE_OUTER_BOUND('',#6617,.T.);
#5434=FACE_OUTER_BOUND('',#6618,.T.);
#5435=FACE_OUTER_BOUND('',#6619,.T.);
#5436=FACE_OUTER_BOUND('',#6620,.T.);
#5437=FACE_OUTER_BOUND('',#6621,.T.);
#5438=FACE_OUTER_BOUND('',#6622,.T.);
#5439=FACE_OUTER_BOUND('',#6626,.T.);
#5440=FACE_OUTER_BOUND('',#6627,.T.);
#5441=FACE_OUTER_BOUND('',#6629,.T.);
#5442=FACE_OUTER_BOUND('',#6630,.T.);
#5443=FACE_OUTER_BOUND('',#6631,.T.);
#5444=FACE_OUTER_BOUND('',#6632,.T.);
#5445=FACE_OUTER_BOUND('',#6633,.T.);
#5446=FACE_OUTER_BOUND('',#6634,.T.);
#5447=FACE_OUTER_BOUND('',#6635,.T.);
#5448=FACE_OUTER_BOUND('',#6636,.T.);
#5449=FACE_OUTER_BOUND('',#6637,.T.);
#5450=FACE_OUTER_BOUND('',#6641,.T.);
#5451=FACE_OUTER_BOUND('',#6642,.T.);
#5452=FACE_OUTER_BOUND('',#6644,.T.);
#5453=FACE_OUTER_BOUND('',#6645,.T.);
#5454=FACE_OUTER_BOUND('',#6646,.T.);
#5455=FACE_OUTER_BOUND('',#6647,.T.);
#5456=FACE_OUTER_BOUND('',#6648,.T.);
#5457=FACE_OUTER_BOUND('',#6649,.T.);
#5458=FACE_OUTER_BOUND('',#6650,.T.);
#5459=FACE_OUTER_BOUND('',#6651,.T.);
#5460=FACE_OUTER_BOUND('',#6652,.T.);
#5461=FACE_OUTER_BOUND('',#6653,.T.);
#5462=FACE_OUTER_BOUND('',#6654,.T.);
#5463=FACE_OUTER_BOUND('',#6658,.T.);
#5464=FACE_OUTER_BOUND('',#6659,.T.);
#5465=FACE_OUTER_BOUND('',#6660,.T.);
#5466=FACE_OUTER_BOUND('',#6661,.T.);
#5467=FACE_OUTER_BOUND('',#6665,.T.);
#5468=FACE_OUTER_BOUND('',#6666,.T.);
#5469=FACE_OUTER_BOUND('',#6667,.T.);
#5470=FACE_OUTER_BOUND('',#6668,.T.);
#5471=FACE_OUTER_BOUND('',#6669,.T.);
#5472=FACE_OUTER_BOUND('',#6670,.T.);
#5473=FACE_OUTER_BOUND('',#6671,.T.);
#5474=FACE_OUTER_BOUND('',#6672,.T.);
#5475=FACE_OUTER_BOUND('',#6673,.T.);
#5476=FACE_OUTER_BOUND('',#6678,.T.);
#5477=FACE_OUTER_BOUND('',#6679,.T.);
#5478=FACE_OUTER_BOUND('',#6680,.T.);
#5479=FACE_OUTER_BOUND('',#6681,.T.);
#5480=FACE_OUTER_BOUND('',#6682,.T.);
#5481=FACE_OUTER_BOUND('',#6683,.T.);
#5482=FACE_OUTER_BOUND('',#6684,.T.);
#5483=FACE_OUTER_BOUND('',#6685,.T.);
#5484=FACE_OUTER_BOUND('',#6686,.T.);
#5485=FACE_OUTER_BOUND('',#6691,.T.);
#5486=FACE_OUTER_BOUND('',#6692,.T.);
#5487=FACE_OUTER_BOUND('',#6693,.T.);
#5488=FACE_OUTER_BOUND('',#6694,.T.);
#5489=FACE_OUTER_BOUND('',#6695,.T.);
#5490=FACE_OUTER_BOUND('',#6696,.T.);
#5491=FACE_OUTER_BOUND('',#6697,.T.);
#5492=FACE_OUTER_BOUND('',#6698,.T.);
#5493=FACE_OUTER_BOUND('',#6699,.T.);
#5494=FACE_OUTER_BOUND('',#6700,.T.);
#5495=FACE_OUTER_BOUND('',#6701,.T.);
#5496=FACE_OUTER_BOUND('',#6702,.T.);
#5497=FACE_OUTER_BOUND('',#6703,.T.);
#5498=FACE_OUTER_BOUND('',#6704,.T.);
#5499=FACE_OUTER_BOUND('',#6705,.T.);
#5500=FACE_OUTER_BOUND('',#6706,.T.);
#5501=FACE_OUTER_BOUND('',#6707,.T.);
#5502=FACE_OUTER_BOUND('',#6708,.T.);
#5503=FACE_OUTER_BOUND('',#6709,.T.);
#5504=FACE_OUTER_BOUND('',#6710,.T.);
#5505=FACE_OUTER_BOUND('',#6711,.T.);
#5506=FACE_OUTER_BOUND('',#6712,.T.);
#5507=FACE_OUTER_BOUND('',#6713,.T.);
#5508=FACE_OUTER_BOUND('',#6714,.T.);
#5509=FACE_OUTER_BOUND('',#6715,.T.);
#5510=FACE_OUTER_BOUND('',#6716,.T.);
#5511=FACE_OUTER_BOUND('',#6717,.T.);
#5512=FACE_OUTER_BOUND('',#6718,.T.);
#5513=FACE_OUTER_BOUND('',#6719,.T.);
#5514=FACE_OUTER_BOUND('',#6720,.T.);
#5515=FACE_OUTER_BOUND('',#6721,.T.);
#5516=FACE_OUTER_BOUND('',#6722,.T.);
#5517=FACE_OUTER_BOUND('',#6723,.T.);
#5518=FACE_OUTER_BOUND('',#6724,.T.);
#5519=FACE_OUTER_BOUND('',#6725,.T.);
#5520=FACE_OUTER_BOUND('',#6726,.T.);
#5521=FACE_OUTER_BOUND('',#6727,.T.);
#5522=FACE_OUTER_BOUND('',#6728,.T.);
#5523=FACE_OUTER_BOUND('',#6729,.T.);
#5524=FACE_OUTER_BOUND('',#6730,.T.);
#5525=FACE_OUTER_BOUND('',#6731,.T.);
#5526=FACE_OUTER_BOUND('',#6732,.T.);
#5527=FACE_OUTER_BOUND('',#6733,.T.);
#5528=FACE_OUTER_BOUND('',#6734,.T.);
#5529=FACE_OUTER_BOUND('',#6735,.T.);
#5530=FACE_OUTER_BOUND('',#6736,.T.);
#5531=FACE_OUTER_BOUND('',#6737,.T.);
#5532=FACE_OUTER_BOUND('',#6738,.T.);
#5533=FACE_OUTER_BOUND('',#6739,.T.);
#5534=FACE_OUTER_BOUND('',#6740,.T.);
#5535=FACE_OUTER_BOUND('',#6741,.T.);
#5536=FACE_OUTER_BOUND('',#6742,.T.);
#6539=EDGE_LOOP('',(#14571,#14572,#14573,#14574));
#6540=EDGE_LOOP('',(#14575,#14576,#14577,#14578));
#6541=EDGE_LOOP('',(#14579,#14580,#14581,#14582));
#6542=EDGE_LOOP('',(#14583,#14584,#14585,#14586));
#6543=EDGE_LOOP('',(#14587,#14588,#14589,#14590));
#6544=EDGE_LOOP('',(#14591,#14592,#14593,#14594));
#6545=EDGE_LOOP('',(#14595,#14596,#14597,#14598,#14599,#14600));
#6546=EDGE_LOOP('',(#14601,#14602,#14603,#14604));
#6547=EDGE_LOOP('',(#14605,#14606,#14607,#14608));
#6548=EDGE_LOOP('',(#14609,#14610,#14611,#14612));
#6549=EDGE_LOOP('',(#14613,#14614,#14615,#14616));
#6550=EDGE_LOOP('',(#14617,#14618,#14619,#14620));
#6551=EDGE_LOOP('',(#14621,#14622,#14623,#14624));
#6552=EDGE_LOOP('',(#14625,#14626,#14627,#14628));
#6553=EDGE_LOOP('',(#14629,#14630,#14631,#14632,#14633,#14634));
#6554=EDGE_LOOP('',(#14635,#14636,#14637,#14638));
#6555=EDGE_LOOP('',(#14639,#14640,#14641,#14642));
#6556=EDGE_LOOP('',(#14643,#14644,#14645,#14646));
#6557=EDGE_LOOP('',(#14647,#14648,#14649,#14650,#14651));
#6558=EDGE_LOOP('',(#14652,#14653,#14654,#14655));
#6559=EDGE_LOOP('',(#14656,#14657,#14658,#14659));
#6560=EDGE_LOOP('',(#14660,#14661,#14662,#14663));
#6561=EDGE_LOOP('',(#14664,#14665,#14666,#14667));
#6562=EDGE_LOOP('',(#14668,#14669,#14670,#14671));
#6563=EDGE_LOOP('',(#14672,#14673,#14674,#14675));
#6564=EDGE_LOOP('',(#14676,#14677,#14678,#14679,#14680,#14681));
#6565=EDGE_LOOP('',(#14682,#14683,#14684,#14685));
#6566=EDGE_LOOP('',(#14686,#14687,#14688));
#6567=EDGE_LOOP('',(#14689,#14690,#14691,#14692));
#6568=EDGE_LOOP('',(#14693,#14694,#14695,#14696,#14697,#14698,#14699,#14700,
#14701,#14702,#14703,#14704));
#6569=EDGE_LOOP('',(#14705,#14706,#14707,#14708));
#6570=EDGE_LOOP('',(#14709,#14710,#14711,#14712));
#6571=EDGE_LOOP('',(#14713,#14714,#14715,#14716));
#6572=EDGE_LOOP('',(#14717,#14718,#14719));
#6573=EDGE_LOOP('',(#14720,#14721,#14722,#14723));
#6574=EDGE_LOOP('',(#14724,#14725,#14726,#14727));
#6575=EDGE_LOOP('',(#14728,#14729,#14730,#14731));
#6576=EDGE_LOOP('',(#14732,#14733,#14734,#14735));
#6577=EDGE_LOOP('',(#14736,#14737,#14738,#14739));
#6578=EDGE_LOOP('',(#14740,#14741,#14742,#14743));
#6579=EDGE_LOOP('',(#14744,#14745,#14746,#14747));
#6580=EDGE_LOOP('',(#14748,#14749,#14750,#14751));
#6581=EDGE_LOOP('',(#14752,#14753,#14754));
#6582=EDGE_LOOP('',(#14755,#14756,#14757,#14758));
#6583=EDGE_LOOP('',(#14759,#14760,#14761,#14762));
#6584=EDGE_LOOP('',(#14763,#14764,#14765,#14766));
#6585=EDGE_LOOP('',(#14767,#14768,#14769,#14770));
#6586=EDGE_LOOP('',(#14771,#14772,#14773,#14774));
#6587=EDGE_LOOP('',(#14775,#14776,#14777,#14778));
#6588=EDGE_LOOP('',(#14779,#14780,#14781,#14782));
#6589=EDGE_LOOP('',(#14783,#14784,#14785,#14786));
#6590=EDGE_LOOP('',(#14787,#14788,#14789,#14790));
#6591=EDGE_LOOP('',(#14791,#14792,#14793,#14794));
#6592=EDGE_LOOP('',(#14795,#14796,#14797,#14798));
#6593=EDGE_LOOP('',(#14799,#14800,#14801,#14802));
#6594=EDGE_LOOP('',(#14803,#14804,#14805,#14806));
#6595=EDGE_LOOP('',(#14807,#14808,#14809));
#6596=EDGE_LOOP('',(#14810,#14811,#14812,#14813));
#6597=EDGE_LOOP('',(#14814,#14815,#14816,#14817));
#6598=EDGE_LOOP('',(#14818,#14819,#14820,#14821));
#6599=EDGE_LOOP('',(#14822,#14823,#14824,#14825));
#6600=EDGE_LOOP('',(#14826,#14827,#14828,#14829));
#6601=EDGE_LOOP('',(#14830,#14831,#14832,#14833));
#6602=EDGE_LOOP('',(#14834,#14835,#14836,#14837));
#6603=EDGE_LOOP('',(#14838,#14839,#14840,#14841,#14842,#14843));
#6604=EDGE_LOOP('',(#14844,#14845,#14846,#14847));
#6605=EDGE_LOOP('',(#14848,#14849,#14850,#14851));
#6606=EDGE_LOOP('',(#14852,#14853,#14854,#14855));
#6607=EDGE_LOOP('',(#14856,#14857,#14858,#14859));
#6608=EDGE_LOOP('',(#14860,#14861,#14862,#14863));
#6609=EDGE_LOOP('',(#14864,#14865,#14866,#14867));
#6610=EDGE_LOOP('',(#14868,#14869,#14870,#14871));
#6611=EDGE_LOOP('',(#14872,#14873,#14874,#14875));
#6612=EDGE_LOOP('',(#14876,#14877,#14878,#14879));
#6613=EDGE_LOOP('',(#14880,#14881,#14882,#14883));
#6614=EDGE_LOOP('',(#14884,#14885,#14886,#14887));
#6615=EDGE_LOOP('',(#14888,#14889,#14890,#14891));
#6616=EDGE_LOOP('',(#14892,#14893,#14894,#14895));
#6617=EDGE_LOOP('',(#14896,#14897,#14898,#14899));
#6618=EDGE_LOOP('',(#14900,#14901,#14902,#14903));
#6619=EDGE_LOOP('',(#14904,#14905,#14906,#14907));
#6620=EDGE_LOOP('',(#14908,#14909,#14910,#14911));
#6621=EDGE_LOOP('',(#14912,#14913,#14914,#14915));
#6622=EDGE_LOOP('',(#14916,#14917,#14918,#14919,#14920,#14921,#14922,#14923));
#6623=EDGE_LOOP('',(#14924));
#6624=EDGE_LOOP('',(#14925));
#6625=EDGE_LOOP('',(#14926));
#6626=EDGE_LOOP('',(#14927,#14928,#14929,#14930,#14931));
#6627=EDGE_LOOP('',(#14932));
#6628=EDGE_LOOP('',(#14933));
#6629=EDGE_LOOP('',(#14934,#14935,#14936,#14937,#14938));
#6630=EDGE_LOOP('',(#14939,#14940,#14941,#14942));
#6631=EDGE_LOOP('',(#14943,#14944,#14945,#14946));
#6632=EDGE_LOOP('',(#14947,#14948,#14949,#14950));
#6633=EDGE_LOOP('',(#14951,#14952,#14953,#14954));
#6634=EDGE_LOOP('',(#14955,#14956,#14957,#14958));
#6635=EDGE_LOOP('',(#14959,#14960,#14961,#14962));
#6636=EDGE_LOOP('',(#14963,#14964,#14965,#14966));
#6637=EDGE_LOOP('',(#14967,#14968,#14969,#14970,#14971,#14972,#14973,#14974));
#6638=EDGE_LOOP('',(#14975));
#6639=EDGE_LOOP('',(#14976));
#6640=EDGE_LOOP('',(#14977));
#6641=EDGE_LOOP('',(#14978,#14979,#14980,#14981,#14982));
#6642=EDGE_LOOP('',(#14983));
#6643=EDGE_LOOP('',(#14984));
#6644=EDGE_LOOP('',(#14985,#14986,#14987,#14988,#14989));
#6645=EDGE_LOOP('',(#14990,#14991,#14992,#14993,#14994));
#6646=EDGE_LOOP('',(#14995,#14996,#14997,#14998,#14999,#15000));
#6647=EDGE_LOOP('',(#15001,#15002,#15003,#15004,#15005));
#6648=EDGE_LOOP('',(#15006,#15007,#15008,#15009,#15010));
#6649=EDGE_LOOP('',(#15011,#15012,#15013,#15014,#15015,#15016));
#6650=EDGE_LOOP('',(#15017,#15018,#15019,#15020,#15021));
#6651=EDGE_LOOP('',(#15022,#15023,#15024,#15025,#15026));
#6652=EDGE_LOOP('',(#15027,#15028,#15029,#15030,#15031,#15032));
#6653=EDGE_LOOP('',(#15033,#15034,#15035,#15036,#15037));
#6654=EDGE_LOOP('',(#15038,#15039,#15040,#15041,#15042,#15043,#15044,#15045,
#15046,#15047,#15048));
#6655=EDGE_LOOP('',(#15049));
#6656=EDGE_LOOP('',(#15050));
#6657=EDGE_LOOP('',(#15051));
#6658=EDGE_LOOP('',(#15052,#15053,#15054,#15055,#15056));
#6659=EDGE_LOOP('',(#15057,#15058,#15059,#15060,#15061,#15062));
#6660=EDGE_LOOP('',(#15063,#15064,#15065,#15066,#15067));
#6661=EDGE_LOOP('',(#15068,#15069,#15070,#15071,#15072,#15073,#15074,#15075,
#15076,#15077,#15078));
#6662=EDGE_LOOP('',(#15079));
#6663=EDGE_LOOP('',(#15080));
#6664=EDGE_LOOP('',(#15081));
#6665=EDGE_LOOP('',(#15082,#15083,#15084,#15085,#15086));
#6666=EDGE_LOOP('',(#15087,#15088,#15089,#15090,#15091,#15092));
#6667=EDGE_LOOP('',(#15093,#15094,#15095,#15096,#15097));
#6668=EDGE_LOOP('',(#15098,#15099,#15100,#15101,#15102));
#6669=EDGE_LOOP('',(#15103,#15104,#15105,#15106,#15107,#15108));
#6670=EDGE_LOOP('',(#15109,#15110,#15111,#15112,#15113));
#6671=EDGE_LOOP('',(#15114,#15115,#15116,#15117,#15118));
#6672=EDGE_LOOP('',(#15119,#15120,#15121,#15122,#15123,#15124));
#6673=EDGE_LOOP('',(#15125,#15126,#15127,#15128,#15129,#15130,#15131,#15132,
#15133,#15134));
#6674=EDGE_LOOP('',(#15135));
#6675=EDGE_LOOP('',(#15136,#15137,#15138,#15139));
#6676=EDGE_LOOP('',(#15140,#15141,#15142,#15143));
#6677=EDGE_LOOP('',(#15144));
#6678=EDGE_LOOP('',(#15145,#15146,#15147,#15148,#15149,#15150));
#6679=EDGE_LOOP('',(#15151,#15152,#15153,#15154));
#6680=EDGE_LOOP('',(#15155,#15156,#15157,#15158,#15159,#15160));
#6681=EDGE_LOOP('',(#15161,#15162,#15163,#15164));
#6682=EDGE_LOOP('',(#15165,#15166,#15167,#15168));
#6683=EDGE_LOOP('',(#15169,#15170,#15171,#15172));
#6684=EDGE_LOOP('',(#15173,#15174,#15175,#15176));
#6685=EDGE_LOOP('',(#15177,#15178,#15179,#15180,#15181));
#6686=EDGE_LOOP('',(#15182,#15183,#15184,#15185,#15186,#15187));
#6687=EDGE_LOOP('',(#15188,#15189,#15190,#15191,#15192,#15193,#15194,#15195));
#6688=EDGE_LOOP('',(#15196,#15197,#15198,#15199,#15200,#15201,#15202,#15203));
#6689=EDGE_LOOP('',(#15204));
#6690=EDGE_LOOP('',(#15205));
#6691=EDGE_LOOP('',(#15206,#15207,#15208,#15209));
#6692=EDGE_LOOP('',(#15210,#15211,#15212,#15213));
#6693=EDGE_LOOP('',(#15214,#15215,#15216,#15217));
#6694=EDGE_LOOP('',(#15218,#15219,#15220,#15221));
#6695=EDGE_LOOP('',(#15222,#15223,#15224,#15225,#15226));
#6696=EDGE_LOOP('',(#15227,#15228,#15229,#15230,#15231,#15232));
#6697=EDGE_LOOP('',(#15233,#15234,#15235,#15236,#15237));
#6698=EDGE_LOOP('',(#15238,#15239,#15240,#15241));
#6699=EDGE_LOOP('',(#15242,#15243,#15244,#15245));
#6700=EDGE_LOOP('',(#15246,#15247,#15248,#15249));
#6701=EDGE_LOOP('',(#15250,#15251,#15252,#15253));
#6702=EDGE_LOOP('',(#15254,#15255,#15256,#15257));
#6703=EDGE_LOOP('',(#15258,#15259,#15260,#15261));
#6704=EDGE_LOOP('',(#15262,#15263,#15264,#15265));
#6705=EDGE_LOOP('',(#15266,#15267,#15268,#15269));
#6706=EDGE_LOOP('',(#15270,#15271,#15272,#15273));
#6707=EDGE_LOOP('',(#15274,#15275,#15276,#15277));
#6708=EDGE_LOOP('',(#15278,#15279,#15280,#15281));
#6709=EDGE_LOOP('',(#15282,#15283,#15284,#15285));
#6710=EDGE_LOOP('',(#15286,#15287,#15288,#15289));
#6711=EDGE_LOOP('',(#15290,#15291,#15292,#15293));
#6712=EDGE_LOOP('',(#15294,#15295,#15296,#15297));
#6713=EDGE_LOOP('',(#15298,#15299,#15300,#15301));
#6714=EDGE_LOOP('',(#15302,#15303,#15304,#15305));
#6715=EDGE_LOOP('',(#15306,#15307,#15308,#15309));
#6716=EDGE_LOOP('',(#15310,#15311,#15312,#15313));
#6717=EDGE_LOOP('',(#15314,#15315,#15316,#15317));
#6718=EDGE_LOOP('',(#15318,#15319,#15320,#15321,#15322,#15323));
#6719=EDGE_LOOP('',(#15324,#15325,#15326,#15327));
#6720=EDGE_LOOP('',(#15328,#15329,#15330,#15331,#15332,#15333,#15334,#15335,
#15336,#15337,#15338,#15339,#15340,#15341));
#6721=EDGE_LOOP('',(#15342,#15343,#15344,#15345));
#6722=EDGE_LOOP('',(#15346,#15347,#15348,#15349,#15350,#15351));
#6723=EDGE_LOOP('',(#15352,#15353,#15354,#15355,#15356,#15357));
#6724=EDGE_LOOP('',(#15358,#15359,#15360,#15361));
#6725=EDGE_LOOP('',(#15362,#15363,#15364,#15365,#15366,#15367));
#6726=EDGE_LOOP('',(#15368,#15369,#15370,#15371));
#6727=EDGE_LOOP('',(#15372,#15373,#15374,#15375));
#6728=EDGE_LOOP('',(#15376,#15377,#15378,#15379,#15380,#15381));
#6729=EDGE_LOOP('',(#15382,#15383,#15384,#15385));
#6730=EDGE_LOOP('',(#15386,#15387,#15388,#15389,#15390,#15391,#15392,#15393,
#15394,#15395,#15396,#15397,#15398,#15399));
#6731=EDGE_LOOP('',(#15400,#15401,#15402,#15403));
#6732=EDGE_LOOP('',(#15404,#15405,#15406,#15407,#15408,#15409));
#6733=EDGE_LOOP('',(#15410,#15411,#15412,#15413,#15414,#15415));
#6734=EDGE_LOOP('',(#15416,#15417,#15418,#15419));
#6735=EDGE_LOOP('',(#15420,#15421,#15422,#15423,#15424,#15425));
#6736=EDGE_LOOP('',(#15426,#15427,#15428,#15429));
#6737=EDGE_LOOP('',(#15430,#15431,#15432,#15433));
#6738=EDGE_LOOP('',(#15434,#15435,#15436,#15437));
#6739=EDGE_LOOP('',(#15438,#15439,#15440,#15441));
#6740=EDGE_LOOP('',(#15442,#15443,#15444,#15445));
#6741=EDGE_LOOP('',(#15446,#15447,#15448,#15449,#15450));
#6742=EDGE_LOOP('',(#15451,#15452,#15453,#15454));
#7685=B_SPLINE_CURVE_WITH_KNOTS('',3,(#60150,#60151,#60152,#60153,#60154,
#60155,#60156,#60157,#60158,#60159,#60160,#60161,#60162,#60163,#60164,#60165),
 .UNSPECIFIED.,.F.,.F.,(4,2,2,2,2,2,2,4),(0.272063574481699,0.273032221187168,
0.283104685038129,0.293177148889091,0.303249612740052,0.323878507973205,
0.334192955589781,0.334675296855046),.UNSPECIFIED.);
#7686=B_SPLINE_CURVE_WITH_KNOTS('',3,(#60212,#60213,#60214,#60215,#60216,
#60217,#60218,#60219,#60220,#60221,#60222,#60223,#60224,#60225,#60226,#60227),
 .UNSPECIFIED.,.F.,.F.,(4,2,2,2,2,2,2,4),(0.0707623923472314,0.0712447336124956,
0.0815591812290722,0.102188076462226,0.112260540313187,0.122333004164148,
0.13240546801511,0.13337411472058),.UNSPECIFIED.);
#7687=B_SPLINE_CURVE_WITH_KNOTS('',3,(#60390,#60391,#60392,#60393,#60394,
#60395,#60396,#60397,#60398,#60399,#60400,#60401,#60402,#60403,#60404,#60405,
#60406,#60407,#60408,#60409,#60410,#60411,#60412,#60413,#60414,#60415,#60416,
#60417),.UNSPECIFIED.,.F.,.F.,(4,3,3,3,3,3,3,3,3,4),(-0.0655070673051713,
-0.055900414383695,-0.0509627360763416,-0.0429749138091241,-0.0358530951083412,
-0.0278292322065516,-0.0195094227834791,-0.00979725211699082,0.,0.000308517528353623),
 .UNSPECIFIED.);
#7688=B_SPLINE_CURVE_WITH_KNOTS('',3,(#60508,#60509,#60510,#60511,#60512,
#60513,#60514,#60515,#60516,#60517,#60518,#60519,#60520,#60521,#60522,#60523,
#60524,#60525,#60526,#60527,#60528,#60529,#60530,#60531,#60532,#60533,#60534,
#60535),.UNSPECIFIED.,.F.,.F.,(4,3,3,3,3,3,3,3,3,4),(-0.131322652134434,
-0.131014134605989,-0.121216882489304,-0.111504711823152,-0.10288152233867,
-0.0951610394988666,-0.0866179312032352,-0.0800513985314073,-0.0695209906596313,
-0.0655070673030884),.UNSPECIFIED.);
#7689=B_SPLINE_CURVE_WITH_KNOTS('',3,(#60582,#60583,#60584,#60585,#60586,
#60587,#60588,#60589,#60590,#60591,#60592,#60593,#60594,#60595,#60596,#60597,
#60598,#60599,#60600,#60601,#60602,#60603,#60604,#60605,#60606,#60607,#60608,
#60609),.UNSPECIFIED.,.F.,.F.,(4,3,3,3,3,3,3,3,3,4),(-0.131322652140315,
-0.13101413461217,-0.121216882493846,-0.111504711827276,-0.102881522342513,
-0.0951610395023411,-0.0866179312064961,-0.0800513985342769,-0.0695209906621001,
-0.0655070673053875),.UNSPECIFIED.);
#7690=B_SPLINE_CURVE_WITH_KNOTS('',3,(#60667,#60668,#60669,#60670,#60671,
#60672,#60673,#60674,#60675,#60676,#60677,#60678,#60679,#60680,#60681,#60682,
#60683,#60684,#60685,#60686,#60687,#60688,#60689,#60690,#60691,#60692,#60693,
#60694),.UNSPECIFIED.,.F.,.F.,(4,3,3,3,3,3,3,3,3,4),(-0.000308517528449134,
0.,0.00979725211682612,0.0195094227831066,0.0281326122676244,0.0358530951076058,
0.0443962034033454,0.050962736075265,0.0614931439471759,0.0655070673037764),
 .UNSPECIFIED.);
#8551=VERTEX_POINT('',#60102);
#8552=VERTEX_POINT('',#60103);
#8553=VERTEX_POINT('',#60105);
#8554=VERTEX_POINT('',#60107);
#8555=VERTEX_POINT('',#60111);
#8556=VERTEX_POINT('',#60113);
#8557=VERTEX_POINT('',#60117);
#8558=VERTEX_POINT('',#60119);
#8559=VERTEX_POINT('',#60126);
#8560=VERTEX_POINT('',#60128);
#8561=VERTEX_POINT('',#60132);
#8562=VERTEX_POINT('',#60136);
#8563=VERTEX_POINT('',#60137);
#8564=VERTEX_POINT('',#60139);
#8565=VERTEX_POINT('',#60141);
#8566=VERTEX_POINT('',#60143);
#8567=VERTEX_POINT('',#60145);
#8568=VERTEX_POINT('',#60149);
#8569=VERTEX_POINT('',#60166);
#8570=VERTEX_POINT('',#60170);
#8571=VERTEX_POINT('',#60171);
#8572=VERTEX_POINT('',#60173);
#8573=VERTEX_POINT('',#60178);
#8574=VERTEX_POINT('',#60179);
#8575=VERTEX_POINT('',#60191);
#8576=VERTEX_POINT('',#60192);
#8577=VERTEX_POINT('',#60194);
#8578=VERTEX_POINT('',#60196);
#8579=VERTEX_POINT('',#60198);
#8580=VERTEX_POINT('',#60200);
#8581=VERTEX_POINT('',#60204);
#8582=VERTEX_POINT('',#60206);
#8583=VERTEX_POINT('',#60210);
#8584=VERTEX_POINT('',#60211);
#8585=VERTEX_POINT('',#60228);
#8586=VERTEX_POINT('',#60230);
#8587=VERTEX_POINT('',#60234);
#8588=VERTEX_POINT('',#60236);
#8589=VERTEX_POINT('',#60238);
#8590=VERTEX_POINT('',#60242);
#8591=VERTEX_POINT('',#60243);
#8592=VERTEX_POINT('',#60245);
#8593=VERTEX_POINT('',#60247);
#8594=VERTEX_POINT('',#60251);
#8595=VERTEX_POINT('',#60253);
#8596=VERTEX_POINT('',#60257);
#8597=VERTEX_POINT('',#60259);
#8598=VERTEX_POINT('',#60266);
#8599=VERTEX_POINT('',#60268);
#8600=VERTEX_POINT('',#60272);
#8601=VERTEX_POINT('',#60276);
#8602=VERTEX_POINT('',#60278);
#8603=VERTEX_POINT('',#60280);
#8604=VERTEX_POINT('',#60282);
#8605=VERTEX_POINT('',#60286);
#8606=VERTEX_POINT('',#60288);
#8607=VERTEX_POINT('',#60292);
#8608=VERTEX_POINT('',#60296);
#8609=VERTEX_POINT('',#60298);
#8610=VERTEX_POINT('',#60300);
#8611=VERTEX_POINT('',#60302);
#8612=VERTEX_POINT('',#60304);
#8613=VERTEX_POINT('',#60306);
#8614=VERTEX_POINT('',#60308);
#8615=VERTEX_POINT('',#60310);
#8616=VERTEX_POINT('',#60312);
#8617=VERTEX_POINT('',#60314);
#8618=VERTEX_POINT('',#60318);
#8619=VERTEX_POINT('',#60322);
#8620=VERTEX_POINT('',#60327);
#8621=VERTEX_POINT('',#60332);
#8622=VERTEX_POINT('',#60337);
#8623=VERTEX_POINT('',#60339);
#8624=VERTEX_POINT('',#60343);
#8625=VERTEX_POINT('',#60347);
#8626=VERTEX_POINT('',#60351);
#8627=VERTEX_POINT('',#60353);
#8628=VERTEX_POINT('',#60357);
#8629=VERTEX_POINT('',#60359);
#8630=VERTEX_POINT('',#60363);
#8631=VERTEX_POINT('',#60364);
#8632=VERTEX_POINT('',#60366);
#8633=VERTEX_POINT('',#60368);
#8634=VERTEX_POINT('',#60372);
#8635=VERTEX_POINT('',#60378);
#8636=VERTEX_POINT('',#60386);
#8637=VERTEX_POINT('',#60388);
#8638=VERTEX_POINT('',#60422);
#8639=VERTEX_POINT('',#60426);
#8640=VERTEX_POINT('',#60430);
#8641=VERTEX_POINT('',#60434);
#8642=VERTEX_POINT('',#60438);
#8643=VERTEX_POINT('',#60446);
#8644=VERTEX_POINT('',#60450);
#8645=VERTEX_POINT('',#60452);
#8646=VERTEX_POINT('',#60456);
#8647=VERTEX_POINT('',#60460);
#8648=VERTEX_POINT('',#60464);
#8649=VERTEX_POINT('',#60466);
#8650=VERTEX_POINT('',#60470);
#8651=VERTEX_POINT('',#60471);
#8652=VERTEX_POINT('',#60473);
#8653=VERTEX_POINT('',#60478);
#8654=VERTEX_POINT('',#60479);
#8655=VERTEX_POINT('',#60491);
#8656=VERTEX_POINT('',#60493);
#8657=VERTEX_POINT('',#60498);
#8658=VERTEX_POINT('',#60499);
#8659=VERTEX_POINT('',#60504);
#8660=VERTEX_POINT('',#60506);
#8661=VERTEX_POINT('',#60537);
#8662=VERTEX_POINT('',#60539);
#8663=VERTEX_POINT('',#60543);
#8664=VERTEX_POINT('',#60545);
#8665=VERTEX_POINT('',#60549);
#8666=VERTEX_POINT('',#60556);
#8667=VERTEX_POINT('',#60560);
#8668=VERTEX_POINT('',#60564);
#8669=VERTEX_POINT('',#60568);
#8670=VERTEX_POINT('',#60574);
#8671=VERTEX_POINT('',#60578);
#8672=VERTEX_POINT('',#60580);
#8673=VERTEX_POINT('',#60613);
#8674=VERTEX_POINT('',#60617);
#8675=VERTEX_POINT('',#60623);
#8676=VERTEX_POINT('',#60625);
#8677=VERTEX_POINT('',#60627);
#8678=VERTEX_POINT('',#60630);
#8679=VERTEX_POINT('',#60632);
#8680=VERTEX_POINT('',#60634);
#8681=VERTEX_POINT('',#60638);
#8682=VERTEX_POINT('',#60641);
#8683=VERTEX_POINT('',#60645);
#8684=VERTEX_POINT('',#60647);
#8685=VERTEX_POINT('',#60653);
#8686=VERTEX_POINT('',#60657);
#8687=VERTEX_POINT('',#60661);
#8688=VERTEX_POINT('',#60665);
#8689=VERTEX_POINT('',#60698);
#8690=VERTEX_POINT('',#60700);
#8691=VERTEX_POINT('',#60702);
#8692=VERTEX_POINT('',#60705);
#8693=VERTEX_POINT('',#60707);
#8694=VERTEX_POINT('',#60709);
#8695=VERTEX_POINT('',#60713);
#8696=VERTEX_POINT('',#60716);
#8697=VERTEX_POINT('',#60720);
#8698=VERTEX_POINT('',#60722);
#8699=VERTEX_POINT('',#60726);
#8700=VERTEX_POINT('',#60728);
#8701=VERTEX_POINT('',#60734);
#8702=VERTEX_POINT('',#60736);
#8703=VERTEX_POINT('',#60740);
#8704=VERTEX_POINT('',#60742);
#8705=VERTEX_POINT('',#60748);
#8706=VERTEX_POINT('',#60750);
#8707=VERTEX_POINT('',#60754);
#8708=VERTEX_POINT('',#60755);
#8709=VERTEX_POINT('',#60760);
#8710=VERTEX_POINT('',#60764);
#8711=VERTEX_POINT('',#60767);
#8712=VERTEX_POINT('',#60769);
#8713=VERTEX_POINT('',#60773);
#8714=VERTEX_POINT('',#60774);
#8715=VERTEX_POINT('',#60779);
#8716=VERTEX_POINT('',#60784);
#8717=VERTEX_POINT('',#60787);
#8718=VERTEX_POINT('',#60789);
#8719=VERTEX_POINT('',#60793);
#8720=VERTEX_POINT('',#60794);
#8721=VERTEX_POINT('',#60801);
#8722=VERTEX_POINT('',#60803);
#8723=VERTEX_POINT('',#60807);
#8724=VERTEX_POINT('',#60808);
#8725=VERTEX_POINT('',#60815);
#8726=VERTEX_POINT('',#60817);
#8727=VERTEX_POINT('',#60819);
#8728=VERTEX_POINT('',#60823);
#8729=VERTEX_POINT('',#60824);
#8730=VERTEX_POINT('',#60829);
#8731=VERTEX_POINT('',#60830);
#8732=VERTEX_POINT('',#60834);
#8733=VERTEX_POINT('',#60837);
#8734=VERTEX_POINT('',#60839);
#8735=VERTEX_POINT('',#60840);
#8736=VERTEX_POINT('',#60842);
#8737=VERTEX_POINT('',#60844);
#8738=VERTEX_POINT('',#60847);
#8739=VERTEX_POINT('',#60848);
#8740=VERTEX_POINT('',#60850);
#8741=VERTEX_POINT('',#60852);
#8742=VERTEX_POINT('',#60856);
#8743=VERTEX_POINT('',#60861);
#8744=VERTEX_POINT('',#60867);
#8745=VERTEX_POINT('',#60871);
#8746=VERTEX_POINT('',#60878);
#8747=VERTEX_POINT('',#60882);
#8748=VERTEX_POINT('',#60884);
#8749=VERTEX_POINT('',#60886);
#8750=VERTEX_POINT('',#60889);
#8751=VERTEX_POINT('',#60890);
#8752=VERTEX_POINT('',#60892);
#8753=VERTEX_POINT('',#60894);
#8754=VERTEX_POINT('',#60896);
#8755=VERTEX_POINT('',#60898);
#8756=VERTEX_POINT('',#60900);
#8757=VERTEX_POINT('',#60902);
#8758=VERTEX_POINT('',#60905);
#8759=VERTEX_POINT('',#60906);
#8760=VERTEX_POINT('',#60908);
#8761=VERTEX_POINT('',#60910);
#8762=VERTEX_POINT('',#60912);
#8763=VERTEX_POINT('',#60914);
#8764=VERTEX_POINT('',#60916);
#8765=VERTEX_POINT('',#60918);
#8766=VERTEX_POINT('',#60921);
#8767=VERTEX_POINT('',#60931);
#8768=VERTEX_POINT('',#60933);
#8769=VERTEX_POINT('',#60937);
#8770=VERTEX_POINT('',#60939);
#8771=VERTEX_POINT('',#60945);
#8772=VERTEX_POINT('',#60947);
#8773=VERTEX_POINT('',#60951);
#8774=VERTEX_POINT('',#60955);
#8775=VERTEX_POINT('',#60961);
#8776=VERTEX_POINT('',#60963);
#8777=VERTEX_POINT('',#60967);
#8778=VERTEX_POINT('',#60976);
#8779=VERTEX_POINT('',#60982);
#8780=VERTEX_POINT('',#60984);
#8781=VERTEX_POINT('',#60988);
#8782=VERTEX_POINT('',#60992);
#8783=VERTEX_POINT('',#60998);
#8784=VERTEX_POINT('',#61000);
#8785=VERTEX_POINT('',#61004);
#8786=VERTEX_POINT('',#61013);
#8787=VERTEX_POINT('',#61019);
#8788=VERTEX_POINT('',#61020);
#8789=VERTEX_POINT('',#61022);
#8790=VERTEX_POINT('',#61024);
#8791=VERTEX_POINT('',#61026);
#8792=VERTEX_POINT('',#61028);
#8793=VERTEX_POINT('',#61032);
#8794=VERTEX_POINT('',#61034);
#8795=VERTEX_POINT('',#61038);
#8796=VERTEX_POINT('',#61040);
#8797=VERTEX_POINT('',#61042);
#8798=VERTEX_POINT('',#61049);
#8799=VERTEX_POINT('',#61051);
#8800=VERTEX_POINT('',#61053);
#8801=VERTEX_POINT('',#61057);
#8802=VERTEX_POINT('',#61058);
#8803=VERTEX_POINT('',#61071);
#8804=VERTEX_POINT('',#61072);
#8805=VERTEX_POINT('',#61074);
#8806=VERTEX_POINT('',#61076);
#8807=VERTEX_POINT('',#61078);
#8808=VERTEX_POINT('',#61080);
#8809=VERTEX_POINT('',#61084);
#8810=VERTEX_POINT('',#61086);
#8811=VERTEX_POINT('',#61090);
#8812=VERTEX_POINT('',#61092);
#8813=VERTEX_POINT('',#61094);
#8814=VERTEX_POINT('',#61101);
#8815=VERTEX_POINT('',#61103);
#8816=VERTEX_POINT('',#61105);
#8817=VERTEX_POINT('',#61109);
#8818=VERTEX_POINT('',#61110);
#10760=EDGE_CURVE('',#8551,#8552,#2284,.T.);
#10761=EDGE_CURVE('',#8552,#8553,#1825,.T.);
#10762=EDGE_CURVE('',#8553,#8554,#2285,.T.);
#10763=EDGE_CURVE('',#8554,#8551,#1826,.T.);
#10764=EDGE_CURVE('',#8555,#8553,#2286,.T.);
#10765=EDGE_CURVE('',#8552,#8556,#2287,.T.);
#10766=EDGE_CURVE('',#8555,#8556,#1827,.T.);
#10767=EDGE_CURVE('',#8557,#8551,#2288,.T.);
#10768=EDGE_CURVE('',#8554,#8558,#2289,.T.);
#10769=EDGE_CURVE('',#8558,#8557,#1828,.T.);
#10770=EDGE_CURVE('',#8556,#8557,#2290,.T.);
#10771=EDGE_CURVE('',#8558,#8555,#2291,.T.);
#10772=EDGE_CURVE('',#8559,#8554,#2292,.T.);
#10773=EDGE_CURVE('',#8560,#8559,#2293,.T.);
#10774=EDGE_CURVE('',#8560,#8558,#2294,.T.);
#10775=EDGE_CURVE('',#8561,#8553,#2295,.T.);
#10776=EDGE_CURVE('',#8559,#8561,#2296,.T.);
#10777=EDGE_CURVE('',#8562,#8563,#2297,.T.);
#10778=EDGE_CURVE('',#8564,#8562,#1829,.T.);
#10779=EDGE_CURVE('',#8565,#8564,#2298,.T.);
#10780=EDGE_CURVE('',#8566,#8565,#2299,.T.);
#10781=EDGE_CURVE('',#8567,#8566,#2300,.T.);
#10782=EDGE_CURVE('',#8567,#8563,#2301,.T.);
#10783=EDGE_CURVE('',#8568,#8562,#7685,.F.);
#10784=EDGE_CURVE('',#8563,#8569,#1830,.F.);
#10785=EDGE_CURVE('',#8569,#8568,#2302,.T.);
#10786=EDGE_CURVE('',#8570,#8571,#2303,.T.);
#10787=EDGE_CURVE('',#8571,#8572,#1831,.T.);
#10788=EDGE_CURVE('',#8572,#8560,#2304,.T.);
#10789=EDGE_CURVE('',#8570,#8560,#1832,.T.);
#10790=EDGE_CURVE('',#8573,#8574,#2305,.T.);
#10791=EDGE_CURVE('',#8574,#8559,#1833,.T.);
#10792=EDGE_CURVE('',#8561,#8573,#1834,.T.);
#10793=EDGE_CURVE('',#8574,#8570,#2306,.T.);
#10794=EDGE_CURVE('',#8571,#8573,#2307,.T.);
#10795=EDGE_CURVE('',#8561,#8572,#2308,.T.);
#10796=EDGE_CURVE('',#8572,#8555,#2309,.T.);
#10797=EDGE_CURVE('',#8575,#8576,#2310,.T.);
#10798=EDGE_CURVE('',#8577,#8575,#2311,.T.);
#10799=EDGE_CURVE('',#8577,#8578,#2312,.T.);
#10800=EDGE_CURVE('',#8579,#8578,#2313,.T.);
#10801=EDGE_CURVE('',#8580,#8579,#2314,.T.);
#10802=EDGE_CURVE('',#8576,#8580,#2315,.T.);
#10803=EDGE_CURVE('',#8581,#8575,#1835,.F.);
#10804=EDGE_CURVE('',#8576,#8582,#1836,.F.);
#10805=EDGE_CURVE('',#8582,#8581,#2316,.T.);
#10806=EDGE_CURVE('',#8583,#8584,#7686,.F.);
#10807=EDGE_CURVE('',#8584,#8585,#2317,.T.);
#10808=EDGE_CURVE('',#8585,#8586,#1837,.F.);
#10809=EDGE_CURVE('',#8586,#8583,#2318,.T.);
#10810=EDGE_CURVE('',#8587,#8584,#1838,.F.);
#10811=EDGE_CURVE('',#8588,#8587,#2319,.T.);
#10812=EDGE_CURVE('',#8589,#8588,#2320,.T.);
#10813=EDGE_CURVE('',#8589,#8585,#2321,.T.);
#10814=EDGE_CURVE('',#8590,#8591,#2322,.T.);
#10815=EDGE_CURVE('',#8591,#8592,#1839,.T.);
#10816=EDGE_CURVE('',#8592,#8593,#2323,.T.);
#10817=EDGE_CURVE('',#8593,#8590,#1840,.T.);
#10818=EDGE_CURVE('',#8594,#8592,#2324,.T.);
#10819=EDGE_CURVE('',#8591,#8595,#2325,.T.);
#10820=EDGE_CURVE('',#8594,#8595,#1841,.T.);
#10821=EDGE_CURVE('',#8596,#8590,#2326,.T.);
#10822=EDGE_CURVE('',#8593,#8597,#2327,.T.);
#10823=EDGE_CURVE('',#8597,#8596,#1842,.T.);
#10824=EDGE_CURVE('',#8595,#8596,#2328,.T.);
#10825=EDGE_CURVE('',#8597,#8594,#2329,.T.);
#10826=EDGE_CURVE('',#8598,#8593,#2330,.T.);
#10827=EDGE_CURVE('',#8599,#8598,#2331,.T.);
#10828=EDGE_CURVE('',#8599,#8597,#2332,.T.);
#10829=EDGE_CURVE('',#8600,#8592,#2333,.T.);
#10830=EDGE_CURVE('',#8598,#8600,#2334,.T.);
#10831=EDGE_CURVE('',#8586,#8601,#2335,.T.);
#10832=EDGE_CURVE('',#8602,#8601,#2336,.T.);
#10833=EDGE_CURVE('',#8603,#8602,#2337,.T.);
#10834=EDGE_CURVE('',#8603,#8604,#2338,.T.);
#10835=EDGE_CURVE('',#8583,#8604,#1843,.T.);
#10836=EDGE_CURVE('',#8605,#8579,#540,.T.);
#10837=EDGE_CURVE('',#8579,#8606,#541,.T.);
#10838=EDGE_CURVE('',#8606,#8605,#542,.T.);
#10839=EDGE_CURVE('',#8607,#8580,#1844,.F.);
#10840=EDGE_CURVE('',#8605,#8607,#2339,.T.);
#10841=EDGE_CURVE('',#8607,#8608,#2340,.T.);
#10842=EDGE_CURVE('',#8609,#8605,#2341,.T.);
#10843=EDGE_CURVE('',#8610,#8609,#2342,.T.);
#10844=EDGE_CURVE('',#8611,#8610,#2343,.T.);
#10845=EDGE_CURVE('',#8612,#8611,#2344,.T.);
#10846=EDGE_CURVE('',#8613,#8612,#2345,.T.);
#10847=EDGE_CURVE('',#8614,#8613,#2346,.T.);
#10848=EDGE_CURVE('',#8615,#8614,#2347,.T.);
#10849=EDGE_CURVE('',#8615,#8616,#2348,.T.);
#10850=EDGE_CURVE('',#8617,#8616,#2349,.T.);
#10851=EDGE_CURVE('',#8608,#8617,#2350,.T.);
#10852=EDGE_CURVE('',#8606,#8618,#2351,.T.);
#10853=EDGE_CURVE('',#8618,#8609,#1845,.T.);
#10854=EDGE_CURVE('',#8619,#8578,#1846,.T.);
#10855=EDGE_CURVE('',#8619,#8606,#2352,.T.);
#10856=EDGE_CURVE('',#8614,#8601,#1847,.T.);
#10857=EDGE_CURVE('',#8601,#8620,#2353,.T.);
#10858=EDGE_CURVE('',#8620,#8615,#1848,.T.);
#10859=EDGE_CURVE('',#8602,#8613,#543,.T.);
#10860=EDGE_CURVE('',#8613,#8621,#544,.T.);
#10861=EDGE_CURVE('',#8621,#8602,#545,.T.);
#10862=EDGE_CURVE('',#8620,#8622,#2354,.T.);
#10863=EDGE_CURVE('',#8622,#8623,#1849,.F.);
#10864=EDGE_CURVE('',#8623,#8615,#2355,.T.);
#10865=EDGE_CURVE('',#8623,#8624,#2356,.T.);
#10866=EDGE_CURVE('',#8616,#8624,#2357,.T.);
#10867=EDGE_CURVE('',#8581,#8625,#2358,.T.);
#10868=EDGE_CURVE('',#8625,#8577,#1850,.T.);
#10869=EDGE_CURVE('',#8625,#8626,#2359,.T.);
#10870=EDGE_CURVE('',#8626,#8627,#1851,.T.);
#10871=EDGE_CURVE('',#8627,#8577,#2360,.T.);
#10872=EDGE_CURVE('',#8626,#8628,#2361,.T.);
#10873=EDGE_CURVE('',#8628,#8629,#1852,.T.);
#10874=EDGE_CURVE('',#8629,#8627,#2362,.T.);
#10875=EDGE_CURVE('',#8630,#8631,#2363,.T.);
#10876=EDGE_CURVE('',#8631,#8632,#546,.T.);
#10877=EDGE_CURVE('',#8632,#8633,#2364,.T.);
#10878=EDGE_CURVE('',#8633,#8630,#1853,.T.);
#10879=EDGE_CURVE('',#8633,#8634,#2365,.T.);
#10880=EDGE_CURVE('',#8634,#8610,#1854,.T.);
#10881=EDGE_CURVE('',#8610,#8630,#2366,.T.);
#10882=EDGE_CURVE('',#8612,#8566,#547,.T.);
#10883=EDGE_CURVE('',#8566,#8635,#548,.T.);
#10884=EDGE_CURVE('',#8635,#8612,#549,.T.);
#10885=EDGE_CURVE('',#8611,#8567,#1855,.T.);
#10886=EDGE_CURVE('',#8634,#8567,#2367,.T.);
#10887=EDGE_CURVE('',#8636,#8632,#550,.T.);
#10888=EDGE_CURVE('',#8631,#8637,#551,.T.);
#10889=EDGE_CURVE('',#8637,#8636,#7687,.T.);
#10890=EDGE_CURVE('',#8628,#8636,#2368,.T.);
#10891=EDGE_CURVE('',#8637,#8629,#2369,.T.);
#10892=EDGE_CURVE('',#8627,#8638,#2370,.T.);
#10893=EDGE_CURVE('',#8578,#8638,#2371,.T.);
#10894=EDGE_CURVE('',#8629,#8639,#2372,.T.);
#10895=EDGE_CURVE('',#8638,#8639,#2373,.T.);
#10896=EDGE_CURVE('',#8637,#8640,#2374,.T.);
#10897=EDGE_CURVE('',#8639,#8640,#2375,.T.);
#10898=EDGE_CURVE('',#8631,#8641,#2376,.T.);
#10899=EDGE_CURVE('',#8640,#8641,#552,.T.);
#10900=EDGE_CURVE('',#8630,#8642,#2377,.T.);
#10901=EDGE_CURVE('',#8641,#8642,#2378,.T.);
#10902=EDGE_CURVE('',#8642,#8609,#2379,.T.);
#10903=EDGE_CURVE('',#8635,#8621,#2380,.T.);
#10904=EDGE_CURVE('',#8565,#8643,#1856,.T.);
#10905=EDGE_CURVE('',#8643,#8635,#2381,.T.);
#10906=EDGE_CURVE('',#8644,#8608,#1857,.F.);
#10907=EDGE_CURVE('',#8617,#8645,#553,.T.);
#10908=EDGE_CURVE('',#8645,#8644,#2382,.T.);
#10909=EDGE_CURVE('',#8617,#8646,#554,.T.);
#10910=EDGE_CURVE('',#8646,#8645,#555,.T.);
#10911=EDGE_CURVE('',#8647,#8616,#1858,.T.);
#10912=EDGE_CURVE('',#8647,#8646,#2383,.T.);
#10913=EDGE_CURVE('',#8648,#8589,#1859,.F.);
#10914=EDGE_CURVE('',#8588,#8649,#1860,.F.);
#10915=EDGE_CURVE('',#8649,#8648,#2384,.T.);
#10916=EDGE_CURVE('',#8650,#8651,#2385,.T.);
#10917=EDGE_CURVE('',#8651,#8652,#1861,.T.);
#10918=EDGE_CURVE('',#8652,#8599,#2386,.T.);
#10919=EDGE_CURVE('',#8650,#8599,#1862,.T.);
#10920=EDGE_CURVE('',#8653,#8654,#2387,.T.);
#10921=EDGE_CURVE('',#8654,#8598,#1863,.T.);
#10922=EDGE_CURVE('',#8600,#8653,#1864,.T.);
#10923=EDGE_CURVE('',#8654,#8650,#2388,.T.);
#10924=EDGE_CURVE('',#8651,#8653,#2389,.T.);
#10925=EDGE_CURVE('',#8600,#8652,#2390,.T.);
#10926=EDGE_CURVE('',#8652,#8594,#2391,.T.);
#10927=EDGE_CURVE('',#8655,#8645,#2392,.T.);
#10928=EDGE_CURVE('',#8656,#8655,#2393,.T.);
#10929=EDGE_CURVE('',#8648,#8656,#2394,.T.);
#10930=EDGE_CURVE('',#8644,#8649,#2395,.T.);
#10931=EDGE_CURVE('',#8657,#8658,#556,.T.);
#10932=EDGE_CURVE('',#8658,#8623,#2396,.T.);
#10933=EDGE_CURVE('',#8622,#8657,#2397,.T.);
#10934=EDGE_CURVE('',#8659,#8658,#557,.T.);
#10935=EDGE_CURVE('',#8657,#8660,#558,.T.);
#10936=EDGE_CURVE('',#8660,#8659,#7688,.T.);
#10937=EDGE_CURVE('',#8660,#8661,#2398,.T.);
#10938=EDGE_CURVE('',#8661,#8662,#1865,.T.);
#10939=EDGE_CURVE('',#8662,#8659,#2399,.T.);
#10940=EDGE_CURVE('',#8661,#8663,#2400,.T.);
#10941=EDGE_CURVE('',#8663,#8664,#1866,.T.);
#10942=EDGE_CURVE('',#8664,#8662,#2401,.T.);
#10943=EDGE_CURVE('',#8665,#8589,#2402,.T.);
#10944=EDGE_CURVE('',#8656,#8665,#1867,.T.);
#10945=EDGE_CURVE('',#8663,#8665,#2403,.T.);
#10946=EDGE_CURVE('',#8656,#8664,#2404,.T.);
#10947=EDGE_CURVE('',#8658,#8666,#2405,.T.);
#10948=EDGE_CURVE('',#8624,#8666,#2406,.T.);
#10949=EDGE_CURVE('',#8659,#8667,#2407,.T.);
#10950=EDGE_CURVE('',#8666,#8667,#559,.T.);
#10951=EDGE_CURVE('',#8662,#8668,#2408,.T.);
#10952=EDGE_CURVE('',#8667,#8668,#2409,.T.);
#10953=EDGE_CURVE('',#8664,#8669,#2410,.T.);
#10954=EDGE_CURVE('',#8668,#8669,#2411,.T.);
#10955=EDGE_CURVE('',#8669,#8655,#2412,.T.);
#10956=EDGE_CURVE('',#8618,#8670,#2413,.T.);
#10957=EDGE_CURVE('',#8670,#8642,#1868,.T.);
#10958=EDGE_CURVE('',#8641,#8671,#560,.T.);
#10959=EDGE_CURVE('',#8671,#8672,#561,.T.);
#10960=EDGE_CURVE('',#8672,#8640,#7689,.T.);
#10961=EDGE_CURVE('',#8670,#8671,#2414,.T.);
#10962=EDGE_CURVE('',#8672,#8673,#2415,.T.);
#10963=EDGE_CURVE('',#8673,#8639,#1869,.T.);
#10964=EDGE_CURVE('',#8673,#8674,#2416,.T.);
#10965=EDGE_CURVE('',#8674,#8638,#1870,.T.);
#10966=EDGE_CURVE('',#8674,#8619,#2417,.T.);
#10967=EDGE_CURVE('',#8675,#8675,#562,.T.);
#10968=EDGE_CURVE('',#8676,#8676,#563,.T.);
#10969=EDGE_CURVE('',#8677,#8677,#564,.T.);
#10970=EDGE_CURVE('',#8678,#8678,#565,.T.);
#10971=EDGE_CURVE('',#8678,#8679,#566,.T.);
#10972=EDGE_CURVE('',#8679,#8680,#567,.T.);
#10973=EDGE_CURVE('',#8680,#8679,#568,.T.);
#10974=EDGE_CURVE('',#8681,#8681,#569,.T.);
#10975=EDGE_CURVE('',#8680,#8682,#2418,.T.);
#10976=EDGE_CURVE('',#8682,#8682,#570,.T.);
#10977=EDGE_CURVE('',#8666,#8683,#571,.T.);
#10978=EDGE_CURVE('',#8683,#8684,#2419,.T.);
#10979=EDGE_CURVE('',#8684,#8624,#1871,.T.);
#10980=EDGE_CURVE('',#8684,#8647,#2420,.T.);
#10981=EDGE_CURVE('',#8646,#8685,#2421,.T.);
#10982=EDGE_CURVE('',#8685,#8655,#1872,.T.);
#10983=EDGE_CURVE('',#8685,#8686,#2422,.T.);
#10984=EDGE_CURVE('',#8686,#8669,#1873,.T.);
#10985=EDGE_CURVE('',#8686,#8687,#2423,.T.);
#10986=EDGE_CURVE('',#8687,#8668,#1874,.T.);
#10987=EDGE_CURVE('',#8687,#8688,#2424,.T.);
#10988=EDGE_CURVE('',#8688,#8667,#7690,.T.);
#10989=EDGE_CURVE('',#8688,#8683,#572,.T.);
#10990=EDGE_CURVE('',#8689,#8689,#573,.T.);
#10991=EDGE_CURVE('',#8690,#8690,#574,.T.);
#10992=EDGE_CURVE('',#8691,#8691,#575,.T.);
#10993=EDGE_CURVE('',#8692,#8692,#576,.T.);
#10994=EDGE_CURVE('',#8692,#8693,#577,.T.);
#10995=EDGE_CURVE('',#8693,#8694,#578,.T.);
#10996=EDGE_CURVE('',#8694,#8693,#579,.T.);
#10997=EDGE_CURVE('',#8695,#8695,#580,.T.);
#10998=EDGE_CURVE('',#8694,#8696,#2425,.T.);
#10999=EDGE_CURVE('',#8696,#8696,#581,.T.);
#11000=EDGE_CURVE('',#8695,#8697,#582,.T.);
#11001=EDGE_CURVE('',#8697,#8698,#583,.T.);
#11002=EDGE_CURVE('',#8698,#8697,#584,.T.);
#11003=EDGE_CURVE('',#8698,#8699,#2426,.T.);
#11004=EDGE_CURVE('',#8700,#8699,#585,.T.);
#11005=EDGE_CURVE('',#8699,#8700,#586,.T.);
#11006=EDGE_CURVE('',#8689,#8700,#587,.T.);
#11007=EDGE_CURVE('',#8681,#8701,#588,.T.);
#11008=EDGE_CURVE('',#8701,#8702,#589,.T.);
#11009=EDGE_CURVE('',#8702,#8701,#590,.T.);
#11010=EDGE_CURVE('',#8702,#8703,#2427,.T.);
#11011=EDGE_CURVE('',#8704,#8703,#591,.T.);
#11012=EDGE_CURVE('',#8703,#8704,#592,.T.);
#11013=EDGE_CURVE('',#8675,#8704,#593,.T.);
#11014=EDGE_CURVE('',#8691,#8705,#594,.T.);
#11015=EDGE_CURVE('',#8705,#8706,#595,.T.);
#11016=EDGE_CURVE('',#8706,#8705,#596,.T.);
#11017=EDGE_CURVE('',#8707,#8708,#597,.T.);
#11018=EDGE_CURVE('',#8708,#8707,#598,.T.);
#11019=EDGE_CURVE('',#8708,#8706,#2428,.T.);
#11020=EDGE_CURVE('',#8709,#8709,#599,.T.);
#11021=EDGE_CURVE('',#8709,#8707,#600,.T.);
#11022=EDGE_CURVE('',#8710,#8710,#601,.T.);
#11023=EDGE_CURVE('',#8677,#8711,#602,.T.);
#11024=EDGE_CURVE('',#8711,#8712,#603,.T.);
#11025=EDGE_CURVE('',#8712,#8711,#604,.T.);
#11026=EDGE_CURVE('',#8713,#8714,#605,.T.);
#11027=EDGE_CURVE('',#8714,#8713,#606,.T.);
#11028=EDGE_CURVE('',#8714,#8712,#2429,.T.);
#11029=EDGE_CURVE('',#8715,#8715,#607,.T.);
#11030=EDGE_CURVE('',#8715,#8713,#608,.T.);
#11031=EDGE_CURVE('',#8581,#8569,#2430,.T.);
#11032=EDGE_CURVE('',#8716,#8716,#609,.T.);
#11033=EDGE_CURVE('',#8690,#8717,#610,.T.);
#11034=EDGE_CURVE('',#8717,#8718,#611,.T.);
#11035=EDGE_CURVE('',#8718,#8717,#612,.T.);
#11036=EDGE_CURVE('',#8719,#8720,#613,.T.);
#11037=EDGE_CURVE('',#8720,#8719,#614,.T.);
#11038=EDGE_CURVE('',#8720,#8718,#2431,.T.);
#11039=EDGE_CURVE('',#8710,#8719,#615,.T.);
#11040=EDGE_CURVE('',#8676,#8721,#616,.T.);
#11041=EDGE_CURVE('',#8721,#8722,#617,.T.);
#11042=EDGE_CURVE('',#8722,#8721,#618,.T.);
#11043=EDGE_CURVE('',#8723,#8724,#619,.T.);
#11044=EDGE_CURVE('',#8724,#8723,#620,.T.);
#11045=EDGE_CURVE('',#8724,#8722,#2432,.T.);
#11046=EDGE_CURVE('',#8716,#8723,#621,.T.);
#11047=EDGE_CURVE('',#8725,#8725,#622,.T.);
#11048=EDGE_CURVE('',#8725,#8726,#623,.T.);
#11049=EDGE_CURVE('',#8726,#8727,#624,.T.);
#11050=EDGE_CURVE('',#8727,#8726,#625,.T.);
#11051=EDGE_CURVE('',#8728,#8729,#626,.T.);
#11052=EDGE_CURVE('',#8729,#8728,#627,.T.);
#11053=EDGE_CURVE('',#8729,#8727,#2433,.T.);
#11054=EDGE_CURVE('',#8730,#8731,#2434,.T.);
#11055=EDGE_CURVE('',#8730,#8582,#2435,.T.);
#11056=EDGE_CURVE('',#8644,#8580,#2436,.T.);
#11057=EDGE_CURVE('',#8732,#8587,#2437,.T.);
#11058=EDGE_CURVE('',#8731,#8732,#2438,.T.);
#11059=EDGE_CURVE('',#8733,#8733,#628,.T.);
#11060=EDGE_CURVE('',#8734,#8735,#2439,.T.);
#11061=EDGE_CURVE('',#8736,#8734,#2440,.T.);
#11062=EDGE_CURVE('',#8737,#8736,#2441,.T.);
#11063=EDGE_CURVE('',#8735,#8737,#2442,.T.);
#11064=EDGE_CURVE('',#8738,#8739,#2443,.T.);
#11065=EDGE_CURVE('',#8740,#8738,#2444,.T.);
#11066=EDGE_CURVE('',#8741,#8740,#2445,.T.);
#11067=EDGE_CURVE('',#8739,#8741,#2446,.T.);
#11068=EDGE_CURVE('',#8742,#8564,#2447,.T.);
#11069=EDGE_CURVE('',#8730,#8568,#1875,.T.);
#11070=EDGE_CURVE('',#8731,#8742,#1876,.T.);
#11071=EDGE_CURVE('',#8732,#8743,#1877,.T.);
#11072=EDGE_CURVE('',#8743,#8742,#2448,.T.);
#11073=EDGE_CURVE('',#8604,#8743,#2449,.T.);
#11074=EDGE_CURVE('',#8744,#8742,#2450,.T.);
#11075=EDGE_CURVE('',#8565,#8744,#2451,.T.);
#11076=EDGE_CURVE('',#8745,#8743,#2452,.T.);
#11077=EDGE_CURVE('',#8744,#8745,#2453,.T.);
#11078=EDGE_CURVE('',#8745,#8603,#2454,.T.);
#11079=EDGE_CURVE('',#8746,#8746,#629,.T.);
#11080=EDGE_CURVE('',#8746,#8728,#630,.T.);
#11081=EDGE_CURVE('',#8747,#8643,#2455,.T.);
#11082=EDGE_CURVE('',#8748,#8747,#2456,.T.);
#11083=EDGE_CURVE('',#8749,#8748,#2457,.T.);
#11084=EDGE_CURVE('',#8621,#8749,#2458,.T.);
#11085=EDGE_CURVE('',#8750,#8751,#2459,.T.);
#11086=EDGE_CURVE('',#8751,#8752,#2460,.T.);
#11087=EDGE_CURVE('',#8752,#8753,#2461,.T.);
#11088=EDGE_CURVE('',#8753,#8754,#2462,.T.);
#11089=EDGE_CURVE('',#8754,#8755,#2463,.T.);
#11090=EDGE_CURVE('',#8756,#8755,#2464,.T.);
#11091=EDGE_CURVE('',#8757,#8756,#2465,.T.);
#11092=EDGE_CURVE('',#8750,#8757,#2466,.T.);
#11093=EDGE_CURVE('',#8758,#8759,#2467,.T.);
#11094=EDGE_CURVE('',#8759,#8760,#2468,.T.);
#11095=EDGE_CURVE('',#8760,#8761,#2469,.T.);
#11096=EDGE_CURVE('',#8761,#8762,#2470,.T.);
#11097=EDGE_CURVE('',#8762,#8763,#2471,.T.);
#11098=EDGE_CURVE('',#8764,#8763,#2472,.T.);
#11099=EDGE_CURVE('',#8765,#8764,#2473,.T.);
#11100=EDGE_CURVE('',#8758,#8765,#2474,.T.);
#11101=EDGE_CURVE('',#8766,#8766,#631,.T.);
#11102=EDGE_CURVE('',#8747,#8744,#1878,.T.);
#11103=EDGE_CURVE('',#8748,#8745,#1879,.T.);
#11104=EDGE_CURVE('',#8749,#8603,#1880,.T.);
#11105=EDGE_CURVE('',#8766,#8767,#632,.T.);
#11106=EDGE_CURVE('',#8767,#8768,#633,.T.);
#11107=EDGE_CURVE('',#8768,#8767,#634,.T.);
#11108=EDGE_CURVE('',#8768,#8769,#2475,.T.);
#11109=EDGE_CURVE('',#8770,#8769,#635,.T.);
#11110=EDGE_CURVE('',#8769,#8770,#636,.T.);
#11111=EDGE_CURVE('',#8733,#8770,#637,.T.);
#11112=EDGE_CURVE('',#8739,#8771,#1881,.T.);
#11113=EDGE_CURVE('',#8771,#8772,#2476,.T.);
#11114=EDGE_CURVE('',#8772,#8738,#1882,.T.);
#11115=EDGE_CURVE('',#8773,#8771,#2477,.T.);
#11116=EDGE_CURVE('',#8773,#8741,#1883,.T.);
#11117=EDGE_CURVE('',#8772,#8774,#2478,.T.);
#11118=EDGE_CURVE('',#8774,#8740,#1884,.T.);
#11119=EDGE_CURVE('',#8774,#8773,#2479,.T.);
#11120=EDGE_CURVE('',#8775,#8772,#2480,.T.);
#11121=EDGE_CURVE('',#8776,#8775,#2481,.T.);
#11122=EDGE_CURVE('',#8776,#8774,#2482,.T.);
#11123=EDGE_CURVE('',#8777,#8771,#2483,.T.);
#11124=EDGE_CURVE('',#8775,#8777,#2484,.T.);
#11125=EDGE_CURVE('',#8777,#8758,#638,.F.);
#11126=EDGE_CURVE('',#8765,#8775,#1885,.T.);
#11127=EDGE_CURVE('',#8764,#8776,#1886,.T.);
#11128=EDGE_CURVE('',#8763,#8778,#639,.F.);
#11129=EDGE_CURVE('',#8778,#8776,#2485,.T.);
#11130=EDGE_CURVE('',#8778,#8773,#2486,.T.);
#11131=EDGE_CURVE('',#8735,#8779,#1887,.T.);
#11132=EDGE_CURVE('',#8779,#8780,#2487,.T.);
#11133=EDGE_CURVE('',#8780,#8734,#1888,.T.);
#11134=EDGE_CURVE('',#8781,#8779,#2488,.T.);
#11135=EDGE_CURVE('',#8781,#8737,#1889,.T.);
#11136=EDGE_CURVE('',#8780,#8782,#2489,.T.);
#11137=EDGE_CURVE('',#8782,#8736,#1890,.T.);
#11138=EDGE_CURVE('',#8782,#8781,#2490,.T.);
#11139=EDGE_CURVE('',#8783,#8780,#2491,.T.);
#11140=EDGE_CURVE('',#8784,#8783,#2492,.T.);
#11141=EDGE_CURVE('',#8784,#8782,#2493,.T.);
#11142=EDGE_CURVE('',#8785,#8779,#2494,.T.);
#11143=EDGE_CURVE('',#8783,#8785,#2495,.T.);
#11144=EDGE_CURVE('',#8785,#8750,#640,.F.);
#11145=EDGE_CURVE('',#8757,#8783,#1891,.T.);
#11146=EDGE_CURVE('',#8756,#8784,#1892,.T.);
#11147=EDGE_CURVE('',#8755,#8786,#641,.F.);
#11148=EDGE_CURVE('',#8786,#8784,#2496,.T.);
#11149=EDGE_CURVE('',#8786,#8781,#2497,.T.);
#11150=EDGE_CURVE('',#8787,#8788,#642,.T.);
#11151=EDGE_CURVE('',#8788,#8789,#2498,.T.);
#11152=EDGE_CURVE('',#8789,#8790,#643,.T.);
#11153=EDGE_CURVE('',#8790,#8791,#2499,.T.);
#11154=EDGE_CURVE('',#8791,#8792,#644,.T.);
#11155=EDGE_CURVE('',#8792,#8787,#2500,.T.);
#11156=EDGE_CURVE('',#8792,#8793,#645,.F.);
#11157=EDGE_CURVE('',#8793,#8794,#2501,.T.);
#11158=EDGE_CURVE('',#8794,#8787,#646,.T.);
#11159=EDGE_CURVE('',#8762,#8795,#2502,.T.);
#11160=EDGE_CURVE('',#8796,#8795,#647,.T.);
#11161=EDGE_CURVE('',#8796,#8797,#648,.T.);
#11162=EDGE_CURVE('',#8793,#8797,#2503,.T.);
#11163=EDGE_CURVE('',#8791,#8759,#2504,.T.);
#11164=EDGE_CURVE('',#8760,#8790,#2505,.T.);
#11165=EDGE_CURVE('',#8794,#8798,#2506,.T.);
#11166=EDGE_CURVE('',#8799,#8798,#649,.T.);
#11167=EDGE_CURVE('',#8800,#8799,#650,.T.);
#11168=EDGE_CURVE('',#8788,#8800,#2507,.T.);
#11169=EDGE_CURVE('',#8801,#8802,#651,.T.);
#11170=EDGE_CURVE('',#8802,#8800,#2508,.T.);
#11171=EDGE_CURVE('',#8799,#8796,#2509,.T.);
#11172=EDGE_CURVE('',#8795,#8801,#2510,.T.);
#11173=EDGE_CURVE('',#8802,#8789,#2511,.T.);
#11174=EDGE_CURVE('',#8761,#8801,#2512,.T.);
#11175=EDGE_CURVE('',#8798,#8797,#2513,.T.);
#11176=EDGE_CURVE('',#8803,#8804,#652,.T.);
#11177=EDGE_CURVE('',#8804,#8805,#2514,.T.);
#11178=EDGE_CURVE('',#8805,#8806,#653,.T.);
#11179=EDGE_CURVE('',#8806,#8807,#2515,.T.);
#11180=EDGE_CURVE('',#8807,#8808,#654,.T.);
#11181=EDGE_CURVE('',#8808,#8803,#2516,.T.);
#11182=EDGE_CURVE('',#8808,#8809,#655,.F.);
#11183=EDGE_CURVE('',#8809,#8810,#2517,.T.);
#11184=EDGE_CURVE('',#8810,#8803,#656,.T.);
#11185=EDGE_CURVE('',#8754,#8811,#2518,.T.);
#11186=EDGE_CURVE('',#8812,#8811,#657,.T.);
#11187=EDGE_CURVE('',#8812,#8813,#658,.T.);
#11188=EDGE_CURVE('',#8809,#8813,#2519,.T.);
#11189=EDGE_CURVE('',#8807,#8751,#2520,.T.);
#11190=EDGE_CURVE('',#8752,#8806,#2521,.T.);
#11191=EDGE_CURVE('',#8810,#8814,#2522,.T.);
#11192=EDGE_CURVE('',#8815,#8814,#659,.T.);
#11193=EDGE_CURVE('',#8816,#8815,#660,.T.);
#11194=EDGE_CURVE('',#8804,#8816,#2523,.T.);
#11195=EDGE_CURVE('',#8817,#8818,#661,.T.);
#11196=EDGE_CURVE('',#8818,#8816,#2524,.T.);
#11197=EDGE_CURVE('',#8815,#8812,#2525,.T.);
#11198=EDGE_CURVE('',#8811,#8817,#2526,.T.);
#11199=EDGE_CURVE('',#8818,#8805,#2527,.T.);
#11200=EDGE_CURVE('',#8753,#8817,#2528,.T.);
#11201=EDGE_CURVE('',#8814,#8813,#2529,.T.);
#14571=ORIENTED_EDGE('',*,*,#10760,.T.);
#14572=ORIENTED_EDGE('',*,*,#10761,.T.);
#14573=ORIENTED_EDGE('',*,*,#10762,.T.);
#14574=ORIENTED_EDGE('',*,*,#10763,.T.);
#14575=ORIENTED_EDGE('',*,*,#10764,.T.);
#14576=ORIENTED_EDGE('',*,*,#10761,.F.);
#14577=ORIENTED_EDGE('',*,*,#10765,.T.);
#14578=ORIENTED_EDGE('',*,*,#10766,.F.);
#14579=ORIENTED_EDGE('',*,*,#10767,.T.);
#14580=ORIENTED_EDGE('',*,*,#10763,.F.);
#14581=ORIENTED_EDGE('',*,*,#10768,.T.);
#14582=ORIENTED_EDGE('',*,*,#10769,.T.);
#14583=ORIENTED_EDGE('',*,*,#10770,.T.);
#14584=ORIENTED_EDGE('',*,*,#10769,.F.);
#14585=ORIENTED_EDGE('',*,*,#10771,.T.);
#14586=ORIENTED_EDGE('',*,*,#10766,.T.);
#14587=ORIENTED_EDGE('',*,*,#10768,.F.);
#14588=ORIENTED_EDGE('',*,*,#10772,.F.);
#14589=ORIENTED_EDGE('',*,*,#10773,.F.);
#14590=ORIENTED_EDGE('',*,*,#10774,.T.);
#14591=ORIENTED_EDGE('',*,*,#10762,.F.);
#14592=ORIENTED_EDGE('',*,*,#10775,.F.);
#14593=ORIENTED_EDGE('',*,*,#10776,.F.);
#14594=ORIENTED_EDGE('',*,*,#10772,.T.);
#14595=ORIENTED_EDGE('',*,*,#10777,.F.);
#14596=ORIENTED_EDGE('',*,*,#10778,.F.);
#14597=ORIENTED_EDGE('',*,*,#10779,.F.);
#14598=ORIENTED_EDGE('',*,*,#10780,.F.);
#14599=ORIENTED_EDGE('',*,*,#10781,.F.);
#14600=ORIENTED_EDGE('',*,*,#10782,.T.);
#14601=ORIENTED_EDGE('',*,*,#10760,.F.);
#14602=ORIENTED_EDGE('',*,*,#10767,.F.);
#14603=ORIENTED_EDGE('',*,*,#10770,.F.);
#14604=ORIENTED_EDGE('',*,*,#10765,.F.);
#14605=ORIENTED_EDGE('',*,*,#10783,.T.);
#14606=ORIENTED_EDGE('',*,*,#10777,.T.);
#14607=ORIENTED_EDGE('',*,*,#10784,.T.);
#14608=ORIENTED_EDGE('',*,*,#10785,.T.);
#14609=ORIENTED_EDGE('',*,*,#10786,.T.);
#14610=ORIENTED_EDGE('',*,*,#10787,.T.);
#14611=ORIENTED_EDGE('',*,*,#10788,.T.);
#14612=ORIENTED_EDGE('',*,*,#10789,.F.);
#14613=ORIENTED_EDGE('',*,*,#10790,.T.);
#14614=ORIENTED_EDGE('',*,*,#10791,.T.);
#14615=ORIENTED_EDGE('',*,*,#10776,.T.);
#14616=ORIENTED_EDGE('',*,*,#10792,.T.);
#14617=ORIENTED_EDGE('',*,*,#10773,.T.);
#14618=ORIENTED_EDGE('',*,*,#10791,.F.);
#14619=ORIENTED_EDGE('',*,*,#10793,.T.);
#14620=ORIENTED_EDGE('',*,*,#10789,.T.);
#14621=ORIENTED_EDGE('',*,*,#10794,.T.);
#14622=ORIENTED_EDGE('',*,*,#10792,.F.);
#14623=ORIENTED_EDGE('',*,*,#10795,.T.);
#14624=ORIENTED_EDGE('',*,*,#10787,.F.);
#14625=ORIENTED_EDGE('',*,*,#10764,.F.);
#14626=ORIENTED_EDGE('',*,*,#10796,.F.);
#14627=ORIENTED_EDGE('',*,*,#10795,.F.);
#14628=ORIENTED_EDGE('',*,*,#10775,.T.);
#14629=ORIENTED_EDGE('',*,*,#10797,.F.);
#14630=ORIENTED_EDGE('',*,*,#10798,.F.);
#14631=ORIENTED_EDGE('',*,*,#10799,.T.);
#14632=ORIENTED_EDGE('',*,*,#10800,.F.);
#14633=ORIENTED_EDGE('',*,*,#10801,.F.);
#14634=ORIENTED_EDGE('',*,*,#10802,.F.);
#14635=ORIENTED_EDGE('',*,*,#10790,.F.);
#14636=ORIENTED_EDGE('',*,*,#10794,.F.);
#14637=ORIENTED_EDGE('',*,*,#10786,.F.);
#14638=ORIENTED_EDGE('',*,*,#10793,.F.);
#14639=ORIENTED_EDGE('',*,*,#10803,.T.);
#14640=ORIENTED_EDGE('',*,*,#10797,.T.);
#14641=ORIENTED_EDGE('',*,*,#10804,.T.);
#14642=ORIENTED_EDGE('',*,*,#10805,.T.);
#14643=ORIENTED_EDGE('',*,*,#10806,.T.);
#14644=ORIENTED_EDGE('',*,*,#10807,.T.);
#14645=ORIENTED_EDGE('',*,*,#10808,.T.);
#14646=ORIENTED_EDGE('',*,*,#10809,.T.);
#14647=ORIENTED_EDGE('',*,*,#10807,.F.);
#14648=ORIENTED_EDGE('',*,*,#10810,.F.);
#14649=ORIENTED_EDGE('',*,*,#10811,.F.);
#14650=ORIENTED_EDGE('',*,*,#10812,.F.);
#14651=ORIENTED_EDGE('',*,*,#10813,.T.);
#14652=ORIENTED_EDGE('',*,*,#10814,.T.);
#14653=ORIENTED_EDGE('',*,*,#10815,.T.);
#14654=ORIENTED_EDGE('',*,*,#10816,.T.);
#14655=ORIENTED_EDGE('',*,*,#10817,.T.);
#14656=ORIENTED_EDGE('',*,*,#10818,.T.);
#14657=ORIENTED_EDGE('',*,*,#10815,.F.);
#14658=ORIENTED_EDGE('',*,*,#10819,.T.);
#14659=ORIENTED_EDGE('',*,*,#10820,.F.);
#14660=ORIENTED_EDGE('',*,*,#10821,.T.);
#14661=ORIENTED_EDGE('',*,*,#10817,.F.);
#14662=ORIENTED_EDGE('',*,*,#10822,.T.);
#14663=ORIENTED_EDGE('',*,*,#10823,.T.);
#14664=ORIENTED_EDGE('',*,*,#10824,.T.);
#14665=ORIENTED_EDGE('',*,*,#10823,.F.);
#14666=ORIENTED_EDGE('',*,*,#10825,.T.);
#14667=ORIENTED_EDGE('',*,*,#10820,.T.);
#14668=ORIENTED_EDGE('',*,*,#10822,.F.);
#14669=ORIENTED_EDGE('',*,*,#10826,.F.);
#14670=ORIENTED_EDGE('',*,*,#10827,.F.);
#14671=ORIENTED_EDGE('',*,*,#10828,.T.);
#14672=ORIENTED_EDGE('',*,*,#10816,.F.);
#14673=ORIENTED_EDGE('',*,*,#10829,.F.);
#14674=ORIENTED_EDGE('',*,*,#10830,.F.);
#14675=ORIENTED_EDGE('',*,*,#10826,.T.);
#14676=ORIENTED_EDGE('',*,*,#10809,.F.);
#14677=ORIENTED_EDGE('',*,*,#10831,.T.);
#14678=ORIENTED_EDGE('',*,*,#10832,.F.);
#14679=ORIENTED_EDGE('',*,*,#10833,.F.);
#14680=ORIENTED_EDGE('',*,*,#10834,.T.);
#14681=ORIENTED_EDGE('',*,*,#10835,.F.);
#14682=ORIENTED_EDGE('',*,*,#10814,.F.);
#14683=ORIENTED_EDGE('',*,*,#10821,.F.);
#14684=ORIENTED_EDGE('',*,*,#10824,.F.);
#14685=ORIENTED_EDGE('',*,*,#10819,.F.);
#14686=ORIENTED_EDGE('',*,*,#10836,.T.);
#14687=ORIENTED_EDGE('',*,*,#10837,.T.);
#14688=ORIENTED_EDGE('',*,*,#10838,.T.);
#14689=ORIENTED_EDGE('',*,*,#10839,.T.);
#14690=ORIENTED_EDGE('',*,*,#10801,.T.);
#14691=ORIENTED_EDGE('',*,*,#10836,.F.);
#14692=ORIENTED_EDGE('',*,*,#10840,.T.);
#14693=ORIENTED_EDGE('',*,*,#10841,.F.);
#14694=ORIENTED_EDGE('',*,*,#10840,.F.);
#14695=ORIENTED_EDGE('',*,*,#10842,.F.);
#14696=ORIENTED_EDGE('',*,*,#10843,.F.);
#14697=ORIENTED_EDGE('',*,*,#10844,.F.);
#14698=ORIENTED_EDGE('',*,*,#10845,.F.);
#14699=ORIENTED_EDGE('',*,*,#10846,.F.);
#14700=ORIENTED_EDGE('',*,*,#10847,.F.);
#14701=ORIENTED_EDGE('',*,*,#10848,.F.);
#14702=ORIENTED_EDGE('',*,*,#10849,.T.);
#14703=ORIENTED_EDGE('',*,*,#10850,.F.);
#14704=ORIENTED_EDGE('',*,*,#10851,.F.);
#14705=ORIENTED_EDGE('',*,*,#10838,.F.);
#14706=ORIENTED_EDGE('',*,*,#10852,.T.);
#14707=ORIENTED_EDGE('',*,*,#10853,.T.);
#14708=ORIENTED_EDGE('',*,*,#10842,.T.);
#14709=ORIENTED_EDGE('',*,*,#10837,.F.);
#14710=ORIENTED_EDGE('',*,*,#10800,.T.);
#14711=ORIENTED_EDGE('',*,*,#10854,.F.);
#14712=ORIENTED_EDGE('',*,*,#10855,.T.);
#14713=ORIENTED_EDGE('',*,*,#10848,.T.);
#14714=ORIENTED_EDGE('',*,*,#10856,.T.);
#14715=ORIENTED_EDGE('',*,*,#10857,.T.);
#14716=ORIENTED_EDGE('',*,*,#10858,.T.);
#14717=ORIENTED_EDGE('',*,*,#10859,.T.);
#14718=ORIENTED_EDGE('',*,*,#10860,.T.);
#14719=ORIENTED_EDGE('',*,*,#10861,.T.);
#14720=ORIENTED_EDGE('',*,*,#10847,.T.);
#14721=ORIENTED_EDGE('',*,*,#10859,.F.);
#14722=ORIENTED_EDGE('',*,*,#10832,.T.);
#14723=ORIENTED_EDGE('',*,*,#10856,.F.);
#14724=ORIENTED_EDGE('',*,*,#10862,.T.);
#14725=ORIENTED_EDGE('',*,*,#10863,.T.);
#14726=ORIENTED_EDGE('',*,*,#10864,.T.);
#14727=ORIENTED_EDGE('',*,*,#10858,.F.);
#14728=ORIENTED_EDGE('',*,*,#10864,.F.);
#14729=ORIENTED_EDGE('',*,*,#10865,.T.);
#14730=ORIENTED_EDGE('',*,*,#10866,.F.);
#14731=ORIENTED_EDGE('',*,*,#10849,.F.);
#14732=ORIENTED_EDGE('',*,*,#10798,.T.);
#14733=ORIENTED_EDGE('',*,*,#10803,.F.);
#14734=ORIENTED_EDGE('',*,*,#10867,.T.);
#14735=ORIENTED_EDGE('',*,*,#10868,.T.);
#14736=ORIENTED_EDGE('',*,*,#10869,.T.);
#14737=ORIENTED_EDGE('',*,*,#10870,.T.);
#14738=ORIENTED_EDGE('',*,*,#10871,.T.);
#14739=ORIENTED_EDGE('',*,*,#10868,.F.);
#14740=ORIENTED_EDGE('',*,*,#10872,.T.);
#14741=ORIENTED_EDGE('',*,*,#10873,.T.);
#14742=ORIENTED_EDGE('',*,*,#10874,.T.);
#14743=ORIENTED_EDGE('',*,*,#10870,.F.);
#14744=ORIENTED_EDGE('',*,*,#10875,.T.);
#14745=ORIENTED_EDGE('',*,*,#10876,.T.);
#14746=ORIENTED_EDGE('',*,*,#10877,.T.);
#14747=ORIENTED_EDGE('',*,*,#10878,.T.);
#14748=ORIENTED_EDGE('',*,*,#10879,.T.);
#14749=ORIENTED_EDGE('',*,*,#10880,.T.);
#14750=ORIENTED_EDGE('',*,*,#10881,.T.);
#14751=ORIENTED_EDGE('',*,*,#10878,.F.);
#14752=ORIENTED_EDGE('',*,*,#10882,.T.);
#14753=ORIENTED_EDGE('',*,*,#10883,.T.);
#14754=ORIENTED_EDGE('',*,*,#10884,.T.);
#14755=ORIENTED_EDGE('',*,*,#10781,.T.);
#14756=ORIENTED_EDGE('',*,*,#10882,.F.);
#14757=ORIENTED_EDGE('',*,*,#10845,.T.);
#14758=ORIENTED_EDGE('',*,*,#10885,.T.);
#14759=ORIENTED_EDGE('',*,*,#10886,.T.);
#14760=ORIENTED_EDGE('',*,*,#10885,.F.);
#14761=ORIENTED_EDGE('',*,*,#10844,.T.);
#14762=ORIENTED_EDGE('',*,*,#10880,.F.);
#14763=ORIENTED_EDGE('',*,*,#10887,.T.);
#14764=ORIENTED_EDGE('',*,*,#10876,.F.);
#14765=ORIENTED_EDGE('',*,*,#10888,.T.);
#14766=ORIENTED_EDGE('',*,*,#10889,.T.);
#14767=ORIENTED_EDGE('',*,*,#10890,.T.);
#14768=ORIENTED_EDGE('',*,*,#10889,.F.);
#14769=ORIENTED_EDGE('',*,*,#10891,.T.);
#14770=ORIENTED_EDGE('',*,*,#10873,.F.);
#14771=ORIENTED_EDGE('',*,*,#10871,.F.);
#14772=ORIENTED_EDGE('',*,*,#10892,.T.);
#14773=ORIENTED_EDGE('',*,*,#10893,.F.);
#14774=ORIENTED_EDGE('',*,*,#10799,.F.);
#14775=ORIENTED_EDGE('',*,*,#10874,.F.);
#14776=ORIENTED_EDGE('',*,*,#10894,.T.);
#14777=ORIENTED_EDGE('',*,*,#10895,.F.);
#14778=ORIENTED_EDGE('',*,*,#10892,.F.);
#14779=ORIENTED_EDGE('',*,*,#10891,.F.);
#14780=ORIENTED_EDGE('',*,*,#10896,.T.);
#14781=ORIENTED_EDGE('',*,*,#10897,.F.);
#14782=ORIENTED_EDGE('',*,*,#10894,.F.);
#14783=ORIENTED_EDGE('',*,*,#10888,.F.);
#14784=ORIENTED_EDGE('',*,*,#10898,.T.);
#14785=ORIENTED_EDGE('',*,*,#10899,.F.);
#14786=ORIENTED_EDGE('',*,*,#10896,.F.);
#14787=ORIENTED_EDGE('',*,*,#10875,.F.);
#14788=ORIENTED_EDGE('',*,*,#10900,.T.);
#14789=ORIENTED_EDGE('',*,*,#10901,.F.);
#14790=ORIENTED_EDGE('',*,*,#10898,.F.);
#14791=ORIENTED_EDGE('',*,*,#10881,.F.);
#14792=ORIENTED_EDGE('',*,*,#10843,.T.);
#14793=ORIENTED_EDGE('',*,*,#10902,.F.);
#14794=ORIENTED_EDGE('',*,*,#10900,.F.);
#14795=ORIENTED_EDGE('',*,*,#10860,.F.);
#14796=ORIENTED_EDGE('',*,*,#10846,.T.);
#14797=ORIENTED_EDGE('',*,*,#10884,.F.);
#14798=ORIENTED_EDGE('',*,*,#10903,.T.);
#14799=ORIENTED_EDGE('',*,*,#10883,.F.);
#14800=ORIENTED_EDGE('',*,*,#10780,.T.);
#14801=ORIENTED_EDGE('',*,*,#10904,.T.);
#14802=ORIENTED_EDGE('',*,*,#10905,.T.);
#14803=ORIENTED_EDGE('',*,*,#10906,.T.);
#14804=ORIENTED_EDGE('',*,*,#10851,.T.);
#14805=ORIENTED_EDGE('',*,*,#10907,.T.);
#14806=ORIENTED_EDGE('',*,*,#10908,.T.);
#14807=ORIENTED_EDGE('',*,*,#10907,.F.);
#14808=ORIENTED_EDGE('',*,*,#10909,.T.);
#14809=ORIENTED_EDGE('',*,*,#10910,.T.);
#14810=ORIENTED_EDGE('',*,*,#10909,.F.);
#14811=ORIENTED_EDGE('',*,*,#10850,.T.);
#14812=ORIENTED_EDGE('',*,*,#10911,.F.);
#14813=ORIENTED_EDGE('',*,*,#10912,.T.);
#14814=ORIENTED_EDGE('',*,*,#10913,.T.);
#14815=ORIENTED_EDGE('',*,*,#10812,.T.);
#14816=ORIENTED_EDGE('',*,*,#10914,.T.);
#14817=ORIENTED_EDGE('',*,*,#10915,.T.);
#14818=ORIENTED_EDGE('',*,*,#10916,.T.);
#14819=ORIENTED_EDGE('',*,*,#10917,.T.);
#14820=ORIENTED_EDGE('',*,*,#10918,.T.);
#14821=ORIENTED_EDGE('',*,*,#10919,.F.);
#14822=ORIENTED_EDGE('',*,*,#10920,.T.);
#14823=ORIENTED_EDGE('',*,*,#10921,.T.);
#14824=ORIENTED_EDGE('',*,*,#10830,.T.);
#14825=ORIENTED_EDGE('',*,*,#10922,.T.);
#14826=ORIENTED_EDGE('',*,*,#10827,.T.);
#14827=ORIENTED_EDGE('',*,*,#10921,.F.);
#14828=ORIENTED_EDGE('',*,*,#10923,.T.);
#14829=ORIENTED_EDGE('',*,*,#10919,.T.);
#14830=ORIENTED_EDGE('',*,*,#10924,.T.);
#14831=ORIENTED_EDGE('',*,*,#10922,.F.);
#14832=ORIENTED_EDGE('',*,*,#10925,.T.);
#14833=ORIENTED_EDGE('',*,*,#10917,.F.);
#14834=ORIENTED_EDGE('',*,*,#10818,.F.);
#14835=ORIENTED_EDGE('',*,*,#10926,.F.);
#14836=ORIENTED_EDGE('',*,*,#10925,.F.);
#14837=ORIENTED_EDGE('',*,*,#10829,.T.);
#14838=ORIENTED_EDGE('',*,*,#10908,.F.);
#14839=ORIENTED_EDGE('',*,*,#10927,.F.);
#14840=ORIENTED_EDGE('',*,*,#10928,.F.);
#14841=ORIENTED_EDGE('',*,*,#10929,.F.);
#14842=ORIENTED_EDGE('',*,*,#10915,.F.);
#14843=ORIENTED_EDGE('',*,*,#10930,.F.);
#14844=ORIENTED_EDGE('',*,*,#10920,.F.);
#14845=ORIENTED_EDGE('',*,*,#10924,.F.);
#14846=ORIENTED_EDGE('',*,*,#10916,.F.);
#14847=ORIENTED_EDGE('',*,*,#10923,.F.);
#14848=ORIENTED_EDGE('',*,*,#10931,.T.);
#14849=ORIENTED_EDGE('',*,*,#10932,.T.);
#14850=ORIENTED_EDGE('',*,*,#10863,.F.);
#14851=ORIENTED_EDGE('',*,*,#10933,.T.);
#14852=ORIENTED_EDGE('',*,*,#10934,.T.);
#14853=ORIENTED_EDGE('',*,*,#10931,.F.);
#14854=ORIENTED_EDGE('',*,*,#10935,.T.);
#14855=ORIENTED_EDGE('',*,*,#10936,.T.);
#14856=ORIENTED_EDGE('',*,*,#10937,.T.);
#14857=ORIENTED_EDGE('',*,*,#10938,.T.);
#14858=ORIENTED_EDGE('',*,*,#10939,.T.);
#14859=ORIENTED_EDGE('',*,*,#10936,.F.);
#14860=ORIENTED_EDGE('',*,*,#10940,.T.);
#14861=ORIENTED_EDGE('',*,*,#10941,.T.);
#14862=ORIENTED_EDGE('',*,*,#10942,.T.);
#14863=ORIENTED_EDGE('',*,*,#10938,.F.);
#14864=ORIENTED_EDGE('',*,*,#10943,.T.);
#14865=ORIENTED_EDGE('',*,*,#10913,.F.);
#14866=ORIENTED_EDGE('',*,*,#10929,.T.);
#14867=ORIENTED_EDGE('',*,*,#10944,.T.);
#14868=ORIENTED_EDGE('',*,*,#10945,.T.);
#14869=ORIENTED_EDGE('',*,*,#10944,.F.);
#14870=ORIENTED_EDGE('',*,*,#10946,.T.);
#14871=ORIENTED_EDGE('',*,*,#10941,.F.);
#14872=ORIENTED_EDGE('',*,*,#10932,.F.);
#14873=ORIENTED_EDGE('',*,*,#10947,.T.);
#14874=ORIENTED_EDGE('',*,*,#10948,.F.);
#14875=ORIENTED_EDGE('',*,*,#10865,.F.);
#14876=ORIENTED_EDGE('',*,*,#10934,.F.);
#14877=ORIENTED_EDGE('',*,*,#10949,.T.);
#14878=ORIENTED_EDGE('',*,*,#10950,.F.);
#14879=ORIENTED_EDGE('',*,*,#10947,.F.);
#14880=ORIENTED_EDGE('',*,*,#10939,.F.);
#14881=ORIENTED_EDGE('',*,*,#10951,.T.);
#14882=ORIENTED_EDGE('',*,*,#10952,.F.);
#14883=ORIENTED_EDGE('',*,*,#10949,.F.);
#14884=ORIENTED_EDGE('',*,*,#10942,.F.);
#14885=ORIENTED_EDGE('',*,*,#10953,.T.);
#14886=ORIENTED_EDGE('',*,*,#10954,.F.);
#14887=ORIENTED_EDGE('',*,*,#10951,.F.);
#14888=ORIENTED_EDGE('',*,*,#10946,.F.);
#14889=ORIENTED_EDGE('',*,*,#10928,.T.);
#14890=ORIENTED_EDGE('',*,*,#10955,.F.);
#14891=ORIENTED_EDGE('',*,*,#10953,.F.);
#14892=ORIENTED_EDGE('',*,*,#10956,.T.);
#14893=ORIENTED_EDGE('',*,*,#10957,.T.);
#14894=ORIENTED_EDGE('',*,*,#10902,.T.);
#14895=ORIENTED_EDGE('',*,*,#10853,.F.);
#14896=ORIENTED_EDGE('',*,*,#10899,.T.);
#14897=ORIENTED_EDGE('',*,*,#10958,.T.);
#14898=ORIENTED_EDGE('',*,*,#10959,.T.);
#14899=ORIENTED_EDGE('',*,*,#10960,.T.);
#14900=ORIENTED_EDGE('',*,*,#10961,.T.);
#14901=ORIENTED_EDGE('',*,*,#10958,.F.);
#14902=ORIENTED_EDGE('',*,*,#10901,.T.);
#14903=ORIENTED_EDGE('',*,*,#10957,.F.);
#14904=ORIENTED_EDGE('',*,*,#10897,.T.);
#14905=ORIENTED_EDGE('',*,*,#10960,.F.);
#14906=ORIENTED_EDGE('',*,*,#10962,.T.);
#14907=ORIENTED_EDGE('',*,*,#10963,.T.);
#14908=ORIENTED_EDGE('',*,*,#10895,.T.);
#14909=ORIENTED_EDGE('',*,*,#10963,.F.);
#14910=ORIENTED_EDGE('',*,*,#10964,.T.);
#14911=ORIENTED_EDGE('',*,*,#10965,.T.);
#14912=ORIENTED_EDGE('',*,*,#10893,.T.);
#14913=ORIENTED_EDGE('',*,*,#10965,.F.);
#14914=ORIENTED_EDGE('',*,*,#10966,.T.);
#14915=ORIENTED_EDGE('',*,*,#10854,.T.);
#14916=ORIENTED_EDGE('',*,*,#10959,.F.);
#14917=ORIENTED_EDGE('',*,*,#10961,.F.);
#14918=ORIENTED_EDGE('',*,*,#10956,.F.);
#14919=ORIENTED_EDGE('',*,*,#10852,.F.);
#14920=ORIENTED_EDGE('',*,*,#10855,.F.);
#14921=ORIENTED_EDGE('',*,*,#10966,.F.);
#14922=ORIENTED_EDGE('',*,*,#10964,.F.);
#14923=ORIENTED_EDGE('',*,*,#10962,.F.);
#14924=ORIENTED_EDGE('',*,*,#10967,.F.);
#14925=ORIENTED_EDGE('',*,*,#10968,.F.);
#14926=ORIENTED_EDGE('',*,*,#10969,.F.);
#14927=ORIENTED_EDGE('',*,*,#10970,.T.);
#14928=ORIENTED_EDGE('',*,*,#10971,.T.);
#14929=ORIENTED_EDGE('',*,*,#10972,.T.);
#14930=ORIENTED_EDGE('',*,*,#10973,.T.);
#14931=ORIENTED_EDGE('',*,*,#10971,.F.);
#14932=ORIENTED_EDGE('',*,*,#10970,.F.);
#14933=ORIENTED_EDGE('',*,*,#10974,.F.);
#14934=ORIENTED_EDGE('',*,*,#10973,.F.);
#14935=ORIENTED_EDGE('',*,*,#10975,.T.);
#14936=ORIENTED_EDGE('',*,*,#10976,.F.);
#14937=ORIENTED_EDGE('',*,*,#10975,.F.);
#14938=ORIENTED_EDGE('',*,*,#10972,.F.);
#14939=ORIENTED_EDGE('',*,*,#10948,.T.);
#14940=ORIENTED_EDGE('',*,*,#10977,.T.);
#14941=ORIENTED_EDGE('',*,*,#10978,.T.);
#14942=ORIENTED_EDGE('',*,*,#10979,.T.);
#14943=ORIENTED_EDGE('',*,*,#10980,.T.);
#14944=ORIENTED_EDGE('',*,*,#10911,.T.);
#14945=ORIENTED_EDGE('',*,*,#10866,.T.);
#14946=ORIENTED_EDGE('',*,*,#10979,.F.);
#14947=ORIENTED_EDGE('',*,*,#10910,.F.);
#14948=ORIENTED_EDGE('',*,*,#10981,.T.);
#14949=ORIENTED_EDGE('',*,*,#10982,.T.);
#14950=ORIENTED_EDGE('',*,*,#10927,.T.);
#14951=ORIENTED_EDGE('',*,*,#10955,.T.);
#14952=ORIENTED_EDGE('',*,*,#10982,.F.);
#14953=ORIENTED_EDGE('',*,*,#10983,.T.);
#14954=ORIENTED_EDGE('',*,*,#10984,.T.);
#14955=ORIENTED_EDGE('',*,*,#10954,.T.);
#14956=ORIENTED_EDGE('',*,*,#10984,.F.);
#14957=ORIENTED_EDGE('',*,*,#10985,.T.);
#14958=ORIENTED_EDGE('',*,*,#10986,.T.);
#14959=ORIENTED_EDGE('',*,*,#10952,.T.);
#14960=ORIENTED_EDGE('',*,*,#10986,.F.);
#14961=ORIENTED_EDGE('',*,*,#10987,.T.);
#14962=ORIENTED_EDGE('',*,*,#10988,.T.);
#14963=ORIENTED_EDGE('',*,*,#10989,.T.);
#14964=ORIENTED_EDGE('',*,*,#10977,.F.);
#14965=ORIENTED_EDGE('',*,*,#10950,.T.);
#14966=ORIENTED_EDGE('',*,*,#10988,.F.);
#14967=ORIENTED_EDGE('',*,*,#10978,.F.);
#14968=ORIENTED_EDGE('',*,*,#10989,.F.);
#14969=ORIENTED_EDGE('',*,*,#10987,.F.);
#14970=ORIENTED_EDGE('',*,*,#10985,.F.);
#14971=ORIENTED_EDGE('',*,*,#10983,.F.);
#14972=ORIENTED_EDGE('',*,*,#10981,.F.);
#14973=ORIENTED_EDGE('',*,*,#10912,.F.);
#14974=ORIENTED_EDGE('',*,*,#10980,.F.);
#14975=ORIENTED_EDGE('',*,*,#10990,.F.);
#14976=ORIENTED_EDGE('',*,*,#10991,.F.);
#14977=ORIENTED_EDGE('',*,*,#10992,.F.);
#14978=ORIENTED_EDGE('',*,*,#10993,.T.);
#14979=ORIENTED_EDGE('',*,*,#10994,.T.);
#14980=ORIENTED_EDGE('',*,*,#10995,.T.);
#14981=ORIENTED_EDGE('',*,*,#10996,.T.);
#14982=ORIENTED_EDGE('',*,*,#10994,.F.);
#14983=ORIENTED_EDGE('',*,*,#10993,.F.);
#14984=ORIENTED_EDGE('',*,*,#10997,.F.);
#14985=ORIENTED_EDGE('',*,*,#10996,.F.);
#14986=ORIENTED_EDGE('',*,*,#10998,.T.);
#14987=ORIENTED_EDGE('',*,*,#10999,.F.);
#14988=ORIENTED_EDGE('',*,*,#10998,.F.);
#14989=ORIENTED_EDGE('',*,*,#10995,.F.);
#14990=ORIENTED_EDGE('',*,*,#10997,.T.);
#14991=ORIENTED_EDGE('',*,*,#11000,.T.);
#14992=ORIENTED_EDGE('',*,*,#11001,.T.);
#14993=ORIENTED_EDGE('',*,*,#11002,.T.);
#14994=ORIENTED_EDGE('',*,*,#11000,.F.);
#14995=ORIENTED_EDGE('',*,*,#11002,.F.);
#14996=ORIENTED_EDGE('',*,*,#11003,.T.);
#14997=ORIENTED_EDGE('',*,*,#11004,.F.);
#14998=ORIENTED_EDGE('',*,*,#11005,.F.);
#14999=ORIENTED_EDGE('',*,*,#11003,.F.);
#15000=ORIENTED_EDGE('',*,*,#11001,.F.);
#15001=ORIENTED_EDGE('',*,*,#10990,.T.);
#15002=ORIENTED_EDGE('',*,*,#11006,.T.);
#15003=ORIENTED_EDGE('',*,*,#11004,.T.);
#15004=ORIENTED_EDGE('',*,*,#11005,.T.);
#15005=ORIENTED_EDGE('',*,*,#11006,.F.);
#15006=ORIENTED_EDGE('',*,*,#10974,.T.);
#15007=ORIENTED_EDGE('',*,*,#11007,.T.);
#15008=ORIENTED_EDGE('',*,*,#11008,.T.);
#15009=ORIENTED_EDGE('',*,*,#11009,.T.);
#15010=ORIENTED_EDGE('',*,*,#11007,.F.);
#15011=ORIENTED_EDGE('',*,*,#11009,.F.);
#15012=ORIENTED_EDGE('',*,*,#11010,.T.);
#15013=ORIENTED_EDGE('',*,*,#11011,.F.);
#15014=ORIENTED_EDGE('',*,*,#11012,.F.);
#15015=ORIENTED_EDGE('',*,*,#11010,.F.);
#15016=ORIENTED_EDGE('',*,*,#11008,.F.);
#15017=ORIENTED_EDGE('',*,*,#10967,.T.);
#15018=ORIENTED_EDGE('',*,*,#11013,.T.);
#15019=ORIENTED_EDGE('',*,*,#11011,.T.);
#15020=ORIENTED_EDGE('',*,*,#11012,.T.);
#15021=ORIENTED_EDGE('',*,*,#11013,.F.);
#15022=ORIENTED_EDGE('',*,*,#10992,.T.);
#15023=ORIENTED_EDGE('',*,*,#11014,.T.);
#15024=ORIENTED_EDGE('',*,*,#11015,.T.);
#15025=ORIENTED_EDGE('',*,*,#11016,.T.);
#15026=ORIENTED_EDGE('',*,*,#11014,.F.);
#15027=ORIENTED_EDGE('',*,*,#11017,.F.);
#15028=ORIENTED_EDGE('',*,*,#11018,.F.);
#15029=ORIENTED_EDGE('',*,*,#11019,.T.);
#15030=ORIENTED_EDGE('',*,*,#11015,.F.);
#15031=ORIENTED_EDGE('',*,*,#11016,.F.);
#15032=ORIENTED_EDGE('',*,*,#11019,.F.);
#15033=ORIENTED_EDGE('',*,*,#11020,.T.);
#15034=ORIENTED_EDGE('',*,*,#11021,.T.);
#15035=ORIENTED_EDGE('',*,*,#11017,.T.);
#15036=ORIENTED_EDGE('',*,*,#11018,.T.);
#15037=ORIENTED_EDGE('',*,*,#11021,.F.);
#15038=ORIENTED_EDGE('',*,*,#10857,.F.);
#15039=ORIENTED_EDGE('',*,*,#10831,.F.);
#15040=ORIENTED_EDGE('',*,*,#10808,.F.);
#15041=ORIENTED_EDGE('',*,*,#10813,.F.);
#15042=ORIENTED_EDGE('',*,*,#10943,.F.);
#15043=ORIENTED_EDGE('',*,*,#10945,.F.);
#15044=ORIENTED_EDGE('',*,*,#10940,.F.);
#15045=ORIENTED_EDGE('',*,*,#10937,.F.);
#15046=ORIENTED_EDGE('',*,*,#10935,.F.);
#15047=ORIENTED_EDGE('',*,*,#10933,.F.);
#15048=ORIENTED_EDGE('',*,*,#10862,.F.);
#15049=ORIENTED_EDGE('',*,*,#11022,.F.);
#15050=ORIENTED_EDGE('',*,*,#10999,.T.);
#15051=ORIENTED_EDGE('',*,*,#11020,.F.);
#15052=ORIENTED_EDGE('',*,*,#10969,.T.);
#15053=ORIENTED_EDGE('',*,*,#11023,.T.);
#15054=ORIENTED_EDGE('',*,*,#11024,.T.);
#15055=ORIENTED_EDGE('',*,*,#11025,.T.);
#15056=ORIENTED_EDGE('',*,*,#11023,.F.);
#15057=ORIENTED_EDGE('',*,*,#11026,.F.);
#15058=ORIENTED_EDGE('',*,*,#11027,.F.);
#15059=ORIENTED_EDGE('',*,*,#11028,.T.);
#15060=ORIENTED_EDGE('',*,*,#11024,.F.);
#15061=ORIENTED_EDGE('',*,*,#11025,.F.);
#15062=ORIENTED_EDGE('',*,*,#11028,.F.);
#15063=ORIENTED_EDGE('',*,*,#11029,.T.);
#15064=ORIENTED_EDGE('',*,*,#11030,.T.);
#15065=ORIENTED_EDGE('',*,*,#11026,.T.);
#15066=ORIENTED_EDGE('',*,*,#11027,.T.);
#15067=ORIENTED_EDGE('',*,*,#11030,.F.);
#15068=ORIENTED_EDGE('',*,*,#10867,.F.);
#15069=ORIENTED_EDGE('',*,*,#11031,.T.);
#15070=ORIENTED_EDGE('',*,*,#10784,.F.);
#15071=ORIENTED_EDGE('',*,*,#10782,.F.);
#15072=ORIENTED_EDGE('',*,*,#10886,.F.);
#15073=ORIENTED_EDGE('',*,*,#10879,.F.);
#15074=ORIENTED_EDGE('',*,*,#10877,.F.);
#15075=ORIENTED_EDGE('',*,*,#10887,.F.);
#15076=ORIENTED_EDGE('',*,*,#10890,.F.);
#15077=ORIENTED_EDGE('',*,*,#10872,.F.);
#15078=ORIENTED_EDGE('',*,*,#10869,.F.);
#15079=ORIENTED_EDGE('',*,*,#11032,.F.);
#15080=ORIENTED_EDGE('',*,*,#10976,.T.);
#15081=ORIENTED_EDGE('',*,*,#11029,.F.);
#15082=ORIENTED_EDGE('',*,*,#10991,.T.);
#15083=ORIENTED_EDGE('',*,*,#11033,.T.);
#15084=ORIENTED_EDGE('',*,*,#11034,.T.);
#15085=ORIENTED_EDGE('',*,*,#11035,.T.);
#15086=ORIENTED_EDGE('',*,*,#11033,.F.);
#15087=ORIENTED_EDGE('',*,*,#11036,.F.);
#15088=ORIENTED_EDGE('',*,*,#11037,.F.);
#15089=ORIENTED_EDGE('',*,*,#11038,.T.);
#15090=ORIENTED_EDGE('',*,*,#11034,.F.);
#15091=ORIENTED_EDGE('',*,*,#11035,.F.);
#15092=ORIENTED_EDGE('',*,*,#11038,.F.);
#15093=ORIENTED_EDGE('',*,*,#11022,.T.);
#15094=ORIENTED_EDGE('',*,*,#11039,.T.);
#15095=ORIENTED_EDGE('',*,*,#11036,.T.);
#15096=ORIENTED_EDGE('',*,*,#11037,.T.);
#15097=ORIENTED_EDGE('',*,*,#11039,.F.);
#15098=ORIENTED_EDGE('',*,*,#10968,.T.);
#15099=ORIENTED_EDGE('',*,*,#11040,.T.);
#15100=ORIENTED_EDGE('',*,*,#11041,.T.);
#15101=ORIENTED_EDGE('',*,*,#11042,.T.);
#15102=ORIENTED_EDGE('',*,*,#11040,.F.);
#15103=ORIENTED_EDGE('',*,*,#11043,.F.);
#15104=ORIENTED_EDGE('',*,*,#11044,.F.);
#15105=ORIENTED_EDGE('',*,*,#11045,.T.);
#15106=ORIENTED_EDGE('',*,*,#11041,.F.);
#15107=ORIENTED_EDGE('',*,*,#11042,.F.);
#15108=ORIENTED_EDGE('',*,*,#11045,.F.);
#15109=ORIENTED_EDGE('',*,*,#11032,.T.);
#15110=ORIENTED_EDGE('',*,*,#11046,.T.);
#15111=ORIENTED_EDGE('',*,*,#11043,.T.);
#15112=ORIENTED_EDGE('',*,*,#11044,.T.);
#15113=ORIENTED_EDGE('',*,*,#11046,.F.);
#15114=ORIENTED_EDGE('',*,*,#11047,.T.);
#15115=ORIENTED_EDGE('',*,*,#11048,.T.);
#15116=ORIENTED_EDGE('',*,*,#11049,.T.);
#15117=ORIENTED_EDGE('',*,*,#11050,.T.);
#15118=ORIENTED_EDGE('',*,*,#11048,.F.);
#15119=ORIENTED_EDGE('',*,*,#11051,.F.);
#15120=ORIENTED_EDGE('',*,*,#11052,.F.);
#15121=ORIENTED_EDGE('',*,*,#11053,.T.);
#15122=ORIENTED_EDGE('',*,*,#11049,.F.);
#15123=ORIENTED_EDGE('',*,*,#11050,.F.);
#15124=ORIENTED_EDGE('',*,*,#11053,.F.);
#15125=ORIENTED_EDGE('',*,*,#11054,.F.);
#15126=ORIENTED_EDGE('',*,*,#11055,.T.);
#15127=ORIENTED_EDGE('',*,*,#10804,.F.);
#15128=ORIENTED_EDGE('',*,*,#10802,.T.);
#15129=ORIENTED_EDGE('',*,*,#11056,.F.);
#15130=ORIENTED_EDGE('',*,*,#10930,.T.);
#15131=ORIENTED_EDGE('',*,*,#10914,.F.);
#15132=ORIENTED_EDGE('',*,*,#10811,.T.);
#15133=ORIENTED_EDGE('',*,*,#11057,.F.);
#15134=ORIENTED_EDGE('',*,*,#11058,.F.);
#15135=ORIENTED_EDGE('',*,*,#11059,.F.);
#15136=ORIENTED_EDGE('',*,*,#11060,.F.);
#15137=ORIENTED_EDGE('',*,*,#11061,.F.);
#15138=ORIENTED_EDGE('',*,*,#11062,.F.);
#15139=ORIENTED_EDGE('',*,*,#11063,.F.);
#15140=ORIENTED_EDGE('',*,*,#11064,.F.);
#15141=ORIENTED_EDGE('',*,*,#11065,.F.);
#15142=ORIENTED_EDGE('',*,*,#11066,.F.);
#15143=ORIENTED_EDGE('',*,*,#11067,.F.);
#15144=ORIENTED_EDGE('',*,*,#11047,.F.);
#15145=ORIENTED_EDGE('',*,*,#11068,.T.);
#15146=ORIENTED_EDGE('',*,*,#10778,.T.);
#15147=ORIENTED_EDGE('',*,*,#10783,.F.);
#15148=ORIENTED_EDGE('',*,*,#11069,.F.);
#15149=ORIENTED_EDGE('',*,*,#11054,.T.);
#15150=ORIENTED_EDGE('',*,*,#11070,.T.);
#15151=ORIENTED_EDGE('',*,*,#11058,.T.);
#15152=ORIENTED_EDGE('',*,*,#11071,.T.);
#15153=ORIENTED_EDGE('',*,*,#11072,.T.);
#15154=ORIENTED_EDGE('',*,*,#11070,.F.);
#15155=ORIENTED_EDGE('',*,*,#11057,.T.);
#15156=ORIENTED_EDGE('',*,*,#10810,.T.);
#15157=ORIENTED_EDGE('',*,*,#10806,.F.);
#15158=ORIENTED_EDGE('',*,*,#10835,.T.);
#15159=ORIENTED_EDGE('',*,*,#11073,.T.);
#15160=ORIENTED_EDGE('',*,*,#11071,.F.);
#15161=ORIENTED_EDGE('',*,*,#11068,.F.);
#15162=ORIENTED_EDGE('',*,*,#11074,.F.);
#15163=ORIENTED_EDGE('',*,*,#11075,.F.);
#15164=ORIENTED_EDGE('',*,*,#10779,.T.);
#15165=ORIENTED_EDGE('',*,*,#11072,.F.);
#15166=ORIENTED_EDGE('',*,*,#11076,.F.);
#15167=ORIENTED_EDGE('',*,*,#11077,.F.);
#15168=ORIENTED_EDGE('',*,*,#11074,.T.);
#15169=ORIENTED_EDGE('',*,*,#11073,.F.);
#15170=ORIENTED_EDGE('',*,*,#10834,.F.);
#15171=ORIENTED_EDGE('',*,*,#11078,.F.);
#15172=ORIENTED_EDGE('',*,*,#11076,.T.);
#15173=ORIENTED_EDGE('',*,*,#10841,.T.);
#15174=ORIENTED_EDGE('',*,*,#10906,.F.);
#15175=ORIENTED_EDGE('',*,*,#11056,.T.);
#15176=ORIENTED_EDGE('',*,*,#10839,.F.);
#15177=ORIENTED_EDGE('',*,*,#11079,.T.);
#15178=ORIENTED_EDGE('',*,*,#11080,.T.);
#15179=ORIENTED_EDGE('',*,*,#11051,.T.);
#15180=ORIENTED_EDGE('',*,*,#11052,.T.);
#15181=ORIENTED_EDGE('',*,*,#11080,.F.);
#15182=ORIENTED_EDGE('',*,*,#10905,.F.);
#15183=ORIENTED_EDGE('',*,*,#11081,.F.);
#15184=ORIENTED_EDGE('',*,*,#11082,.F.);
#15185=ORIENTED_EDGE('',*,*,#11083,.F.);
#15186=ORIENTED_EDGE('',*,*,#11084,.F.);
#15187=ORIENTED_EDGE('',*,*,#10903,.F.);
#15188=ORIENTED_EDGE('',*,*,#11085,.T.);
#15189=ORIENTED_EDGE('',*,*,#11086,.T.);
#15190=ORIENTED_EDGE('',*,*,#11087,.T.);
#15191=ORIENTED_EDGE('',*,*,#11088,.T.);
#15192=ORIENTED_EDGE('',*,*,#11089,.T.);
#15193=ORIENTED_EDGE('',*,*,#11090,.F.);
#15194=ORIENTED_EDGE('',*,*,#11091,.F.);
#15195=ORIENTED_EDGE('',*,*,#11092,.F.);
#15196=ORIENTED_EDGE('',*,*,#11093,.T.);
#15197=ORIENTED_EDGE('',*,*,#11094,.T.);
#15198=ORIENTED_EDGE('',*,*,#11095,.T.);
#15199=ORIENTED_EDGE('',*,*,#11096,.T.);
#15200=ORIENTED_EDGE('',*,*,#11097,.T.);
#15201=ORIENTED_EDGE('',*,*,#11098,.F.);
#15202=ORIENTED_EDGE('',*,*,#11099,.F.);
#15203=ORIENTED_EDGE('',*,*,#11100,.F.);
#15204=ORIENTED_EDGE('',*,*,#11101,.F.);
#15205=ORIENTED_EDGE('',*,*,#11079,.F.);
#15206=ORIENTED_EDGE('',*,*,#11082,.T.);
#15207=ORIENTED_EDGE('',*,*,#11102,.T.);
#15208=ORIENTED_EDGE('',*,*,#11077,.T.);
#15209=ORIENTED_EDGE('',*,*,#11103,.F.);
#15210=ORIENTED_EDGE('',*,*,#11081,.T.);
#15211=ORIENTED_EDGE('',*,*,#10904,.F.);
#15212=ORIENTED_EDGE('',*,*,#11075,.T.);
#15213=ORIENTED_EDGE('',*,*,#11102,.F.);
#15214=ORIENTED_EDGE('',*,*,#10861,.F.);
#15215=ORIENTED_EDGE('',*,*,#11084,.T.);
#15216=ORIENTED_EDGE('',*,*,#11104,.T.);
#15217=ORIENTED_EDGE('',*,*,#10833,.T.);
#15218=ORIENTED_EDGE('',*,*,#11078,.T.);
#15219=ORIENTED_EDGE('',*,*,#11104,.F.);
#15220=ORIENTED_EDGE('',*,*,#11083,.T.);
#15221=ORIENTED_EDGE('',*,*,#11103,.T.);
#15222=ORIENTED_EDGE('',*,*,#11101,.T.);
#15223=ORIENTED_EDGE('',*,*,#11105,.T.);
#15224=ORIENTED_EDGE('',*,*,#11106,.T.);
#15225=ORIENTED_EDGE('',*,*,#11107,.T.);
#15226=ORIENTED_EDGE('',*,*,#11105,.F.);
#15227=ORIENTED_EDGE('',*,*,#11107,.F.);
#15228=ORIENTED_EDGE('',*,*,#11108,.T.);
#15229=ORIENTED_EDGE('',*,*,#11109,.F.);
#15230=ORIENTED_EDGE('',*,*,#11110,.F.);
#15231=ORIENTED_EDGE('',*,*,#11108,.F.);
#15232=ORIENTED_EDGE('',*,*,#11106,.F.);
#15233=ORIENTED_EDGE('',*,*,#11059,.T.);
#15234=ORIENTED_EDGE('',*,*,#11111,.T.);
#15235=ORIENTED_EDGE('',*,*,#11109,.T.);
#15236=ORIENTED_EDGE('',*,*,#11110,.T.);
#15237=ORIENTED_EDGE('',*,*,#11111,.F.);
#15238=ORIENTED_EDGE('',*,*,#11064,.T.);
#15239=ORIENTED_EDGE('',*,*,#11112,.T.);
#15240=ORIENTED_EDGE('',*,*,#11113,.T.);
#15241=ORIENTED_EDGE('',*,*,#11114,.T.);
#15242=ORIENTED_EDGE('',*,*,#11115,.T.);
#15243=ORIENTED_EDGE('',*,*,#11112,.F.);
#15244=ORIENTED_EDGE('',*,*,#11067,.T.);
#15245=ORIENTED_EDGE('',*,*,#11116,.F.);
#15246=ORIENTED_EDGE('',*,*,#11065,.T.);
#15247=ORIENTED_EDGE('',*,*,#11114,.F.);
#15248=ORIENTED_EDGE('',*,*,#11117,.T.);
#15249=ORIENTED_EDGE('',*,*,#11118,.T.);
#15250=ORIENTED_EDGE('',*,*,#11066,.T.);
#15251=ORIENTED_EDGE('',*,*,#11118,.F.);
#15252=ORIENTED_EDGE('',*,*,#11119,.T.);
#15253=ORIENTED_EDGE('',*,*,#11116,.T.);
#15254=ORIENTED_EDGE('',*,*,#11117,.F.);
#15255=ORIENTED_EDGE('',*,*,#11120,.F.);
#15256=ORIENTED_EDGE('',*,*,#11121,.F.);
#15257=ORIENTED_EDGE('',*,*,#11122,.T.);
#15258=ORIENTED_EDGE('',*,*,#11113,.F.);
#15259=ORIENTED_EDGE('',*,*,#11123,.F.);
#15260=ORIENTED_EDGE('',*,*,#11124,.F.);
#15261=ORIENTED_EDGE('',*,*,#11120,.T.);
#15262=ORIENTED_EDGE('',*,*,#11124,.T.);
#15263=ORIENTED_EDGE('',*,*,#11125,.T.);
#15264=ORIENTED_EDGE('',*,*,#11100,.T.);
#15265=ORIENTED_EDGE('',*,*,#11126,.T.);
#15266=ORIENTED_EDGE('',*,*,#11121,.T.);
#15267=ORIENTED_EDGE('',*,*,#11126,.F.);
#15268=ORIENTED_EDGE('',*,*,#11099,.T.);
#15269=ORIENTED_EDGE('',*,*,#11127,.T.);
#15270=ORIENTED_EDGE('',*,*,#11098,.T.);
#15271=ORIENTED_EDGE('',*,*,#11128,.T.);
#15272=ORIENTED_EDGE('',*,*,#11129,.T.);
#15273=ORIENTED_EDGE('',*,*,#11127,.F.);
#15274=ORIENTED_EDGE('',*,*,#11119,.F.);
#15275=ORIENTED_EDGE('',*,*,#11122,.F.);
#15276=ORIENTED_EDGE('',*,*,#11129,.F.);
#15277=ORIENTED_EDGE('',*,*,#11130,.T.);
#15278=ORIENTED_EDGE('',*,*,#11060,.T.);
#15279=ORIENTED_EDGE('',*,*,#11131,.T.);
#15280=ORIENTED_EDGE('',*,*,#11132,.T.);
#15281=ORIENTED_EDGE('',*,*,#11133,.T.);
#15282=ORIENTED_EDGE('',*,*,#11134,.T.);
#15283=ORIENTED_EDGE('',*,*,#11131,.F.);
#15284=ORIENTED_EDGE('',*,*,#11063,.T.);
#15285=ORIENTED_EDGE('',*,*,#11135,.F.);
#15286=ORIENTED_EDGE('',*,*,#11061,.T.);
#15287=ORIENTED_EDGE('',*,*,#11133,.F.);
#15288=ORIENTED_EDGE('',*,*,#11136,.T.);
#15289=ORIENTED_EDGE('',*,*,#11137,.T.);
#15290=ORIENTED_EDGE('',*,*,#11062,.T.);
#15291=ORIENTED_EDGE('',*,*,#11137,.F.);
#15292=ORIENTED_EDGE('',*,*,#11138,.T.);
#15293=ORIENTED_EDGE('',*,*,#11135,.T.);
#15294=ORIENTED_EDGE('',*,*,#11136,.F.);
#15295=ORIENTED_EDGE('',*,*,#11139,.F.);
#15296=ORIENTED_EDGE('',*,*,#11140,.F.);
#15297=ORIENTED_EDGE('',*,*,#11141,.T.);
#15298=ORIENTED_EDGE('',*,*,#11132,.F.);
#15299=ORIENTED_EDGE('',*,*,#11142,.F.);
#15300=ORIENTED_EDGE('',*,*,#11143,.F.);
#15301=ORIENTED_EDGE('',*,*,#11139,.T.);
#15302=ORIENTED_EDGE('',*,*,#11143,.T.);
#15303=ORIENTED_EDGE('',*,*,#11144,.T.);
#15304=ORIENTED_EDGE('',*,*,#11092,.T.);
#15305=ORIENTED_EDGE('',*,*,#11145,.T.);
#15306=ORIENTED_EDGE('',*,*,#11140,.T.);
#15307=ORIENTED_EDGE('',*,*,#11145,.F.);
#15308=ORIENTED_EDGE('',*,*,#11091,.T.);
#15309=ORIENTED_EDGE('',*,*,#11146,.T.);
#15310=ORIENTED_EDGE('',*,*,#11090,.T.);
#15311=ORIENTED_EDGE('',*,*,#11147,.T.);
#15312=ORIENTED_EDGE('',*,*,#11148,.T.);
#15313=ORIENTED_EDGE('',*,*,#11146,.F.);
#15314=ORIENTED_EDGE('',*,*,#11138,.F.);
#15315=ORIENTED_EDGE('',*,*,#11141,.F.);
#15316=ORIENTED_EDGE('',*,*,#11148,.F.);
#15317=ORIENTED_EDGE('',*,*,#11149,.T.);
#15318=ORIENTED_EDGE('',*,*,#11150,.T.);
#15319=ORIENTED_EDGE('',*,*,#11151,.T.);
#15320=ORIENTED_EDGE('',*,*,#11152,.T.);
#15321=ORIENTED_EDGE('',*,*,#11153,.T.);
#15322=ORIENTED_EDGE('',*,*,#11154,.T.);
#15323=ORIENTED_EDGE('',*,*,#11155,.T.);
#15324=ORIENTED_EDGE('',*,*,#11155,.F.);
#15325=ORIENTED_EDGE('',*,*,#11156,.T.);
#15326=ORIENTED_EDGE('',*,*,#11157,.T.);
#15327=ORIENTED_EDGE('',*,*,#11158,.T.);
#15328=ORIENTED_EDGE('',*,*,#11115,.F.);
#15329=ORIENTED_EDGE('',*,*,#11130,.F.);
#15330=ORIENTED_EDGE('',*,*,#11128,.F.);
#15331=ORIENTED_EDGE('',*,*,#11097,.F.);
#15332=ORIENTED_EDGE('',*,*,#11159,.T.);
#15333=ORIENTED_EDGE('',*,*,#11160,.F.);
#15334=ORIENTED_EDGE('',*,*,#11161,.T.);
#15335=ORIENTED_EDGE('',*,*,#11162,.F.);
#15336=ORIENTED_EDGE('',*,*,#11156,.F.);
#15337=ORIENTED_EDGE('',*,*,#11154,.F.);
#15338=ORIENTED_EDGE('',*,*,#11163,.T.);
#15339=ORIENTED_EDGE('',*,*,#11093,.F.);
#15340=ORIENTED_EDGE('',*,*,#11125,.F.);
#15341=ORIENTED_EDGE('',*,*,#11123,.T.);
#15342=ORIENTED_EDGE('',*,*,#11153,.F.);
#15343=ORIENTED_EDGE('',*,*,#11164,.F.);
#15344=ORIENTED_EDGE('',*,*,#11094,.F.);
#15345=ORIENTED_EDGE('',*,*,#11163,.F.);
#15346=ORIENTED_EDGE('',*,*,#11150,.F.);
#15347=ORIENTED_EDGE('',*,*,#11158,.F.);
#15348=ORIENTED_EDGE('',*,*,#11165,.T.);
#15349=ORIENTED_EDGE('',*,*,#11166,.F.);
#15350=ORIENTED_EDGE('',*,*,#11167,.F.);
#15351=ORIENTED_EDGE('',*,*,#11168,.F.);
#15352=ORIENTED_EDGE('',*,*,#11169,.T.);
#15353=ORIENTED_EDGE('',*,*,#11170,.T.);
#15354=ORIENTED_EDGE('',*,*,#11167,.T.);
#15355=ORIENTED_EDGE('',*,*,#11171,.T.);
#15356=ORIENTED_EDGE('',*,*,#11160,.T.);
#15357=ORIENTED_EDGE('',*,*,#11172,.T.);
#15358=ORIENTED_EDGE('',*,*,#11151,.F.);
#15359=ORIENTED_EDGE('',*,*,#11168,.T.);
#15360=ORIENTED_EDGE('',*,*,#11170,.F.);
#15361=ORIENTED_EDGE('',*,*,#11173,.T.);
#15362=ORIENTED_EDGE('',*,*,#11152,.F.);
#15363=ORIENTED_EDGE('',*,*,#11173,.F.);
#15364=ORIENTED_EDGE('',*,*,#11169,.F.);
#15365=ORIENTED_EDGE('',*,*,#11174,.F.);
#15366=ORIENTED_EDGE('',*,*,#11095,.F.);
#15367=ORIENTED_EDGE('',*,*,#11164,.T.);
#15368=ORIENTED_EDGE('',*,*,#11172,.F.);
#15369=ORIENTED_EDGE('',*,*,#11159,.F.);
#15370=ORIENTED_EDGE('',*,*,#11096,.F.);
#15371=ORIENTED_EDGE('',*,*,#11174,.T.);
#15372=ORIENTED_EDGE('',*,*,#11171,.F.);
#15373=ORIENTED_EDGE('',*,*,#11166,.T.);
#15374=ORIENTED_EDGE('',*,*,#11175,.T.);
#15375=ORIENTED_EDGE('',*,*,#11161,.F.);
#15376=ORIENTED_EDGE('',*,*,#11176,.T.);
#15377=ORIENTED_EDGE('',*,*,#11177,.T.);
#15378=ORIENTED_EDGE('',*,*,#11178,.T.);
#15379=ORIENTED_EDGE('',*,*,#11179,.T.);
#15380=ORIENTED_EDGE('',*,*,#11180,.T.);
#15381=ORIENTED_EDGE('',*,*,#11181,.T.);
#15382=ORIENTED_EDGE('',*,*,#11181,.F.);
#15383=ORIENTED_EDGE('',*,*,#11182,.T.);
#15384=ORIENTED_EDGE('',*,*,#11183,.T.);
#15385=ORIENTED_EDGE('',*,*,#11184,.T.);
#15386=ORIENTED_EDGE('',*,*,#11134,.F.);
#15387=ORIENTED_EDGE('',*,*,#11149,.F.);
#15388=ORIENTED_EDGE('',*,*,#11147,.F.);
#15389=ORIENTED_EDGE('',*,*,#11089,.F.);
#15390=ORIENTED_EDGE('',*,*,#11185,.T.);
#15391=ORIENTED_EDGE('',*,*,#11186,.F.);
#15392=ORIENTED_EDGE('',*,*,#11187,.T.);
#15393=ORIENTED_EDGE('',*,*,#11188,.F.);
#15394=ORIENTED_EDGE('',*,*,#11182,.F.);
#15395=ORIENTED_EDGE('',*,*,#11180,.F.);
#15396=ORIENTED_EDGE('',*,*,#11189,.T.);
#15397=ORIENTED_EDGE('',*,*,#11085,.F.);
#15398=ORIENTED_EDGE('',*,*,#11144,.F.);
#15399=ORIENTED_EDGE('',*,*,#11142,.T.);
#15400=ORIENTED_EDGE('',*,*,#11179,.F.);
#15401=ORIENTED_EDGE('',*,*,#11190,.F.);
#15402=ORIENTED_EDGE('',*,*,#11086,.F.);
#15403=ORIENTED_EDGE('',*,*,#11189,.F.);
#15404=ORIENTED_EDGE('',*,*,#11176,.F.);
#15405=ORIENTED_EDGE('',*,*,#11184,.F.);
#15406=ORIENTED_EDGE('',*,*,#11191,.T.);
#15407=ORIENTED_EDGE('',*,*,#11192,.F.);
#15408=ORIENTED_EDGE('',*,*,#11193,.F.);
#15409=ORIENTED_EDGE('',*,*,#11194,.F.);
#15410=ORIENTED_EDGE('',*,*,#11195,.T.);
#15411=ORIENTED_EDGE('',*,*,#11196,.T.);
#15412=ORIENTED_EDGE('',*,*,#11193,.T.);
#15413=ORIENTED_EDGE('',*,*,#11197,.T.);
#15414=ORIENTED_EDGE('',*,*,#11186,.T.);
#15415=ORIENTED_EDGE('',*,*,#11198,.T.);
#15416=ORIENTED_EDGE('',*,*,#11177,.F.);
#15417=ORIENTED_EDGE('',*,*,#11194,.T.);
#15418=ORIENTED_EDGE('',*,*,#11196,.F.);
#15419=ORIENTED_EDGE('',*,*,#11199,.T.);
#15420=ORIENTED_EDGE('',*,*,#11178,.F.);
#15421=ORIENTED_EDGE('',*,*,#11199,.F.);
#15422=ORIENTED_EDGE('',*,*,#11195,.F.);
#15423=ORIENTED_EDGE('',*,*,#11200,.F.);
#15424=ORIENTED_EDGE('',*,*,#11087,.F.);
#15425=ORIENTED_EDGE('',*,*,#11190,.T.);
#15426=ORIENTED_EDGE('',*,*,#11198,.F.);
#15427=ORIENTED_EDGE('',*,*,#11185,.F.);
#15428=ORIENTED_EDGE('',*,*,#11088,.F.);
#15429=ORIENTED_EDGE('',*,*,#11200,.T.);
#15430=ORIENTED_EDGE('',*,*,#11197,.F.);
#15431=ORIENTED_EDGE('',*,*,#11192,.T.);
#15432=ORIENTED_EDGE('',*,*,#11201,.T.);
#15433=ORIENTED_EDGE('',*,*,#11187,.F.);
#15434=ORIENTED_EDGE('',*,*,#11183,.F.);
#15435=ORIENTED_EDGE('',*,*,#11188,.T.);
#15436=ORIENTED_EDGE('',*,*,#11201,.F.);
#15437=ORIENTED_EDGE('',*,*,#11191,.F.);
#15438=ORIENTED_EDGE('',*,*,#11157,.F.);
#15439=ORIENTED_EDGE('',*,*,#11162,.T.);
#15440=ORIENTED_EDGE('',*,*,#11175,.F.);
#15441=ORIENTED_EDGE('',*,*,#11165,.F.);
#15442=ORIENTED_EDGE('',*,*,#10771,.F.);
#15443=ORIENTED_EDGE('',*,*,#10774,.F.);
#15444=ORIENTED_EDGE('',*,*,#10788,.F.);
#15445=ORIENTED_EDGE('',*,*,#10796,.T.);
#15446=ORIENTED_EDGE('',*,*,#10785,.F.);
#15447=ORIENTED_EDGE('',*,*,#11031,.F.);
#15448=ORIENTED_EDGE('',*,*,#10805,.F.);
#15449=ORIENTED_EDGE('',*,*,#11055,.F.);
#15450=ORIENTED_EDGE('',*,*,#11069,.T.);
#15451=ORIENTED_EDGE('',*,*,#10825,.F.);
#15452=ORIENTED_EDGE('',*,*,#10828,.F.);
#15453=ORIENTED_EDGE('',*,*,#10918,.F.);
#15454=ORIENTED_EDGE('',*,*,#10926,.T.);
#19293=ADVANCED_FACE('',(#5359),#4671,.T.);
#19294=ADVANCED_FACE('',(#5360),#4672,.T.);
#19295=ADVANCED_FACE('',(#5361),#4673,.T.);
#19296=ADVANCED_FACE('',(#5362),#4674,.T.);
#19297=ADVANCED_FACE('',(#5363),#1399,.F.);
#19298=ADVANCED_FACE('',(#5364),#1400,.F.);
#19299=ADVANCED_FACE('',(#5365,#1717),#1401,.T.);
#19300=ADVANCED_FACE('',(#5366),#4675,.T.);
#19301=ADVANCED_FACE('',(#5367),#4676,.T.);
#19302=ADVANCED_FACE('',(#5368),#4677,.T.);
#19303=ADVANCED_FACE('',(#5369),#4678,.T.);
#19304=ADVANCED_FACE('',(#5370),#4679,.T.);
#19305=ADVANCED_FACE('',(#5371),#1402,.F.);
#19306=ADVANCED_FACE('',(#5372,#1718),#1403,.T.);
#19307=ADVANCED_FACE('',(#5373),#4680,.T.);
#19308=ADVANCED_FACE('',(#5374),#4681,.T.);
#19309=ADVANCED_FACE('',(#5375),#1404,.T.);
#19310=ADVANCED_FACE('',(#5376),#4682,.T.);
#19311=ADVANCED_FACE('',(#5377),#4683,.T.);
#19312=ADVANCED_FACE('',(#5378),#4684,.T.);
#19313=ADVANCED_FACE('',(#5379),#4685,.T.);
#19314=ADVANCED_FACE('',(#5380),#1405,.F.);
#19315=ADVANCED_FACE('',(#5381),#1406,.F.);
#19316=ADVANCED_FACE('',(#5382,#1719),#1407,.T.);
#19317=ADVANCED_FACE('',(#5383),#181,.T.);
#19318=ADVANCED_FACE('',(#5384),#4686,.T.);
#19319=ADVANCED_FACE('',(#5385),#1408,.T.);
#19320=ADVANCED_FACE('',(#5386),#4687,.T.);
#19321=ADVANCED_FACE('',(#5387),#4688,.T.);
#19322=ADVANCED_FACE('',(#5388),#4689,.T.);
#19323=ADVANCED_FACE('',(#5389),#182,.T.);
#19324=ADVANCED_FACE('',(#5390),#4690,.T.);
#19325=ADVANCED_FACE('',(#5391),#4691,.T.);
#19326=ADVANCED_FACE('',(#5392),#1409,.T.);
#19327=ADVANCED_FACE('',(#5393),#4692,.T.);
#19328=ADVANCED_FACE('',(#5394),#4693,.T.);
#19329=ADVANCED_FACE('',(#5395),#4694,.T.);
#19330=ADVANCED_FACE('',(#5396),#4695,.T.);
#19331=ADVANCED_FACE('',(#5397),#4696,.T.);
#19332=ADVANCED_FACE('',(#5398),#183,.T.);
#19333=ADVANCED_FACE('',(#5399),#4697,.T.);
#19334=ADVANCED_FACE('',(#5400),#4698,.T.);
#19335=ADVANCED_FACE('',(#5401),#1215,.T.);
#19336=ADVANCED_FACE('',(#5402),#4699,.T.);
#19337=ADVANCED_FACE('',(#5403),#1410,.T.);
#19338=ADVANCED_FACE('',(#5404),#1411,.T.);
#19339=ADVANCED_FACE('',(#5405),#1412,.T.);
#19340=ADVANCED_FACE('',(#5406),#4700,.T.);
#19341=ADVANCED_FACE('',(#5407),#1413,.T.);
#19342=ADVANCED_FACE('',(#5408),#1414,.T.);
#19343=ADVANCED_FACE('',(#5409),#4701,.T.);
#19344=ADVANCED_FACE('',(#5410),#4702,.T.);
#19345=ADVANCED_FACE('',(#5411),#4703,.T.);
#19346=ADVANCED_FACE('',(#5412),#184,.T.);
#19347=ADVANCED_FACE('',(#5413),#4704,.T.);
#19348=ADVANCED_FACE('',(#5414),#4705,.T.);
#19349=ADVANCED_FACE('',(#5415),#4706,.T.);
#19350=ADVANCED_FACE('',(#5416),#4707,.T.);
#19351=ADVANCED_FACE('',(#5417),#4708,.T.);
#19352=ADVANCED_FACE('',(#5418),#4709,.T.);
#19353=ADVANCED_FACE('',(#5419),#1415,.F.);
#19354=ADVANCED_FACE('',(#5420,#1720),#1416,.F.);
#19355=ADVANCED_FACE('',(#5421),#4710,.T.);
#19356=ADVANCED_FACE('',(#5422),#1216,.T.);
#19357=ADVANCED_FACE('',(#5423),#4711,.T.);
#19358=ADVANCED_FACE('',(#5424),#4712,.T.);
#19359=ADVANCED_FACE('',(#5425),#4713,.T.);
#19360=ADVANCED_FACE('',(#5426),#4714,.T.);
#19361=ADVANCED_FACE('',(#5427),#1417,.T.);
#19362=ADVANCED_FACE('',(#5428),#4715,.T.);
#19363=ADVANCED_FACE('',(#5429),#1418,.T.);
#19364=ADVANCED_FACE('',(#5430),#1419,.T.);
#19365=ADVANCED_FACE('',(#5431),#1420,.T.);
#19366=ADVANCED_FACE('',(#5432),#4716,.T.);
#19367=ADVANCED_FACE('',(#5433),#1217,.T.);
#19368=ADVANCED_FACE('',(#5434),#4717,.T.);
#19369=ADVANCED_FACE('',(#5435),#4718,.T.);
#19370=ADVANCED_FACE('',(#5436),#4719,.T.);
#19371=ADVANCED_FACE('',(#5437),#4720,.T.);
#19372=ADVANCED_FACE('',(#5438,#1721,#1722,#1723),#1421,.T.);
#19373=ADVANCED_FACE('',(#5439),#1218,.T.);
#19374=ADVANCED_FACE('',(#5440,#1724),#1422,.F.);
#19375=ADVANCED_FACE('',(#5441),#4721,.T.);
#19376=ADVANCED_FACE('',(#5442),#4722,.T.);
#19377=ADVANCED_FACE('',(#5443),#4723,.T.);
#19378=ADVANCED_FACE('',(#5444),#4724,.T.);
#19379=ADVANCED_FACE('',(#5445),#4725,.T.);
#19380=ADVANCED_FACE('',(#5446),#4726,.T.);
#19381=ADVANCED_FACE('',(#5447),#4727,.T.);
#19382=ADVANCED_FACE('',(#5448),#1219,.T.);
#19383=ADVANCED_FACE('',(#5449,#1725,#1726,#1727),#1423,.T.);
#19384=ADVANCED_FACE('',(#5450),#1220,.T.);
#19385=ADVANCED_FACE('',(#5451,#1728),#1424,.F.);
#19386=ADVANCED_FACE('',(#5452),#4728,.T.);
#19387=ADVANCED_FACE('',(#5453),#1221,.T.);
#19388=ADVANCED_FACE('',(#5454),#4729,.F.);
#19389=ADVANCED_FACE('',(#5455),#1222,.T.);
#19390=ADVANCED_FACE('',(#5456),#1223,.T.);
#19391=ADVANCED_FACE('',(#5457),#4730,.F.);
#19392=ADVANCED_FACE('',(#5458),#1224,.T.);
#19393=ADVANCED_FACE('',(#5459),#1225,.T.);
#19394=ADVANCED_FACE('',(#5460),#4731,.F.);
#19395=ADVANCED_FACE('',(#5461),#1226,.T.);
#19396=ADVANCED_FACE('',(#5462,#1729,#1730,#1731),#1425,.F.);
#19397=ADVANCED_FACE('',(#5463),#1227,.T.);
#19398=ADVANCED_FACE('',(#5464),#4732,.F.);
#19399=ADVANCED_FACE('',(#5465),#1228,.T.);
#19400=ADVANCED_FACE('',(#5466,#1732,#1733,#1734),#1426,.F.);
#19401=ADVANCED_FACE('',(#5467),#1229,.T.);
#19402=ADVANCED_FACE('',(#5468),#4733,.F.);
#19403=ADVANCED_FACE('',(#5469),#1230,.T.);
#19404=ADVANCED_FACE('',(#5470),#1231,.T.);
#19405=ADVANCED_FACE('',(#5471),#4734,.F.);
#19406=ADVANCED_FACE('',(#5472),#1232,.T.);
#19407=ADVANCED_FACE('',(#5473),#1233,.T.);
#19408=ADVANCED_FACE('',(#5474),#4735,.F.);
#19409=ADVANCED_FACE('',(#5475,#1735,#1736,#1737,#1738),#1427,.T.);
#19410=ADVANCED_FACE('',(#5476),#4736,.T.);
#19411=ADVANCED_FACE('',(#5477),#4737,.T.);
#19412=ADVANCED_FACE('',(#5478),#4738,.T.);
#19413=ADVANCED_FACE('',(#5479),#1428,.T.);
#19414=ADVANCED_FACE('',(#5480),#1429,.T.);
#19415=ADVANCED_FACE('',(#5481),#1430,.T.);
#19416=ADVANCED_FACE('',(#5482),#4739,.T.);
#19417=ADVANCED_FACE('',(#5483),#1234,.T.);
#19418=ADVANCED_FACE('',(#5484,#1739,#1740,#1741,#1742),#1431,.F.);
#19419=ADVANCED_FACE('',(#5485),#4740,.T.);
#19420=ADVANCED_FACE('',(#5486),#4741,.T.);
#19421=ADVANCED_FACE('',(#5487),#4742,.T.);
#19422=ADVANCED_FACE('',(#5488),#4743,.T.);
#19423=ADVANCED_FACE('',(#5489),#1235,.T.);
#19424=ADVANCED_FACE('',(#5490),#4744,.F.);
#19425=ADVANCED_FACE('',(#5491),#1236,.T.);
#19426=ADVANCED_FACE('',(#5492),#4745,.T.);
#19427=ADVANCED_FACE('',(#5493),#4746,.T.);
#19428=ADVANCED_FACE('',(#5494),#4747,.T.);
#19429=ADVANCED_FACE('',(#5495),#4748,.T.);
#19430=ADVANCED_FACE('',(#5496),#1432,.F.);
#19431=ADVANCED_FACE('',(#5497),#1433,.F.);
#19432=ADVANCED_FACE('',(#5498),#4749,.T.);
#19433=ADVANCED_FACE('',(#5499),#4750,.T.);
#19434=ADVANCED_FACE('',(#5500),#4751,.T.);
#19435=ADVANCED_FACE('',(#5501),#1434,.F.);
#19436=ADVANCED_FACE('',(#5502),#4752,.T.);
#19437=ADVANCED_FACE('',(#5503),#4753,.T.);
#19438=ADVANCED_FACE('',(#5504),#4754,.T.);
#19439=ADVANCED_FACE('',(#5505),#4755,.T.);
#19440=ADVANCED_FACE('',(#5506),#1435,.F.);
#19441=ADVANCED_FACE('',(#5507),#1436,.F.);
#19442=ADVANCED_FACE('',(#5508),#4756,.T.);
#19443=ADVANCED_FACE('',(#5509),#4757,.T.);
#19444=ADVANCED_FACE('',(#5510),#4758,.T.);
#19445=ADVANCED_FACE('',(#5511),#1437,.F.);
#19446=ADVANCED_FACE('',(#5512),#4759,.T.);
#19447=ADVANCED_FACE('',(#5513),#4760,.T.);
#19448=ADVANCED_FACE('',(#5514),#1438,.F.);
#19449=ADVANCED_FACE('',(#5515),#1439,.T.);
#19450=ADVANCED_FACE('',(#5516),#1440,.T.);
#19451=ADVANCED_FACE('',(#5517),#4761,.T.);
#19452=ADVANCED_FACE('',(#5518),#1441,.T.);
#19453=ADVANCED_FACE('',(#5519),#1442,.T.);
#19454=ADVANCED_FACE('',(#5520),#1443,.T.);
#19455=ADVANCED_FACE('',(#5521),#4762,.T.);
#19456=ADVANCED_FACE('',(#5522),#4763,.T.);
#19457=ADVANCED_FACE('',(#5523),#4764,.T.);
#19458=ADVANCED_FACE('',(#5524),#1444,.F.);
#19459=ADVANCED_FACE('',(#5525),#1445,.T.);
#19460=ADVANCED_FACE('',(#5526),#1446,.T.);
#19461=ADVANCED_FACE('',(#5527),#4765,.T.);
#19462=ADVANCED_FACE('',(#5528),#1447,.T.);
#19463=ADVANCED_FACE('',(#5529),#1448,.T.);
#19464=ADVANCED_FACE('',(#5530),#1449,.T.);
#19465=ADVANCED_FACE('',(#5531),#4766,.T.);
#19466=ADVANCED_FACE('',(#5532),#1450,.T.);
#19467=ADVANCED_FACE('',(#5533),#1451,.T.);
#19468=ADVANCED_FACE('',(#5534),#1452,.F.);
#19469=ADVANCED_FACE('',(#5535),#1453,.T.);
#19470=ADVANCED_FACE('',(#5536),#1454,.F.);
#20119=CLOSED_SHELL('',(#19293,#19294,#19295,#19296,#19297,#19298,#19299,
#19300,#19301,#19302,#19303,#19304,#19305,#19306,#19307,#19308,#19309,#19310,
#19311,#19312,#19313,#19314,#19315,#19316,#19317,#19318,#19319,#19320,#19321,
#19322,#19323,#19324,#19325,#19326,#19327,#19328,#19329,#19330,#19331,#19332,
#19333,#19334,#19335,#19336,#19337,#19338,#19339,#19340,#19341,#19342,#19343,
#19344,#19345,#19346,#19347,#19348,#19349,#19350,#19351,#19352,#19353,#19354,
#19355,#19356,#19357,#19358,#19359,#19360,#19361,#19362,#19363,#19364,#19365,
#19366,#19367,#19368,#19369,#19370,#19371,#19372,#19373,#19374,#19375,#19376,
#19377,#19378,#19379,#19380,#19381,#19382,#19383,#19384,#19385,#19386,#19387,
#19388,#19389,#19390,#19391,#19392,#19393,#19394,#19395,#19396,#19397,#19398,
#19399,#19400,#19401,#19402,#19403,#19404,#19405,#19406,#19407,#19408,#19409,
#19410,#19411,#19412,#19413,#19414,#19415,#19416,#19417,#19418,#19419,#19420,
#19421,#19422,#19423,#19424,#19425,#19426,#19427,#19428,#19429,#19430,#19431,
#19432,#19433,#19434,#19435,#19436,#19437,#19438,#19439,#19440,#19441,#19442,
#19443,#19444,#19445,#19446,#19447,#19448,#19449,#19450,#19451,#19452,#19453,
#19454,#19455,#19456,#19457,#19458,#19459,#19460,#19461,#19462,#19463,#19464,
#19465,#19466,#19467,#19468,#19469,#19470));
#20892=AXIS2_PLACEMENT_3D('',#60100,#23945,#23946);
#20893=AXIS2_PLACEMENT_3D('',#60101,#23947,#23948);
#20894=AXIS2_PLACEMENT_3D('',#60106,#23950,#23951);
#20895=AXIS2_PLACEMENT_3D('',#60109,#23953,#23954);
#20896=AXIS2_PLACEMENT_3D('',#60110,#23955,#23956);
#20897=AXIS2_PLACEMENT_3D('',#60115,#23959,#23960);
#20898=AXIS2_PLACEMENT_3D('',#60116,#23961,#23962);
#20899=AXIS2_PLACEMENT_3D('',#60121,#23965,#23966);
#20900=AXIS2_PLACEMENT_3D('',#60122,#23967,#23968);
#20901=AXIS2_PLACEMENT_3D('',#60125,#23971,#23972);
#20902=AXIS2_PLACEMENT_3D('',#60131,#23976,#23977);
#20903=AXIS2_PLACEMENT_3D('',#60135,#23980,#23981);
#20904=AXIS2_PLACEMENT_3D('',#60140,#23983,#23984);
#20905=AXIS2_PLACEMENT_3D('',#60148,#23989,#23990);
#20906=AXIS2_PLACEMENT_3D('',#60167,#23991,#23992);
#20907=AXIS2_PLACEMENT_3D('',#60169,#23994,#23995);
#20908=AXIS2_PLACEMENT_3D('',#60174,#23997,#23998);
#20909=AXIS2_PLACEMENT_3D('',#60176,#24000,#24001);
#20910=AXIS2_PLACEMENT_3D('',#60177,#24002,#24003);
#20911=AXIS2_PLACEMENT_3D('',#60181,#24005,#24006);
#20912=AXIS2_PLACEMENT_3D('',#60182,#24007,#24008);
#20913=AXIS2_PLACEMENT_3D('',#60183,#24009,#24010);
#20914=AXIS2_PLACEMENT_3D('',#60185,#24012,#24013);
#20915=AXIS2_PLACEMENT_3D('',#60188,#24016,#24017);
#20916=AXIS2_PLACEMENT_3D('',#60190,#24019,#24020);
#20917=AXIS2_PLACEMENT_3D('',#60203,#24027,#24028);
#20918=AXIS2_PLACEMENT_3D('',#60205,#24029,#24030);
#20919=AXIS2_PLACEMENT_3D('',#60207,#24031,#24032);
#20920=AXIS2_PLACEMENT_3D('',#60209,#24034,#24035);
#20921=AXIS2_PLACEMENT_3D('',#60231,#24037,#24038);
#20922=AXIS2_PLACEMENT_3D('',#60233,#24040,#24041);
#20923=AXIS2_PLACEMENT_3D('',#60235,#24042,#24043);
#20924=AXIS2_PLACEMENT_3D('',#60241,#24047,#24048);
#20925=AXIS2_PLACEMENT_3D('',#60246,#24050,#24051);
#20926=AXIS2_PLACEMENT_3D('',#60249,#24053,#24054);
#20927=AXIS2_PLACEMENT_3D('',#60250,#24055,#24056);
#20928=AXIS2_PLACEMENT_3D('',#60255,#24059,#24060);
#20929=AXIS2_PLACEMENT_3D('',#60256,#24061,#24062);
#20930=AXIS2_PLACEMENT_3D('',#60261,#24065,#24066);
#20931=AXIS2_PLACEMENT_3D('',#60262,#24067,#24068);
#20932=AXIS2_PLACEMENT_3D('',#60265,#24071,#24072);
#20933=AXIS2_PLACEMENT_3D('',#60271,#24076,#24077);
#20934=AXIS2_PLACEMENT_3D('',#60275,#24080,#24081);
#20935=AXIS2_PLACEMENT_3D('',#60284,#24086,#24087);
#20936=AXIS2_PLACEMENT_3D('',#60285,#24088,#24089);
#20937=AXIS2_PLACEMENT_3D('',#60287,#24090,#24091);
#20938=AXIS2_PLACEMENT_3D('',#60289,#24092,#24093);
#20939=AXIS2_PLACEMENT_3D('',#60290,#24094,#24095);
#20940=AXIS2_PLACEMENT_3D('',#60291,#24096,#24097);
#20941=AXIS2_PLACEMENT_3D('',#60293,#24098,#24099);
#20942=AXIS2_PLACEMENT_3D('',#60295,#24101,#24102);
#20943=AXIS2_PLACEMENT_3D('',#60317,#24114,#24115);
#20944=AXIS2_PLACEMENT_3D('',#60320,#24117,#24118);
#20945=AXIS2_PLACEMENT_3D('',#60321,#24119,#24120);
#20946=AXIS2_PLACEMENT_3D('',#60323,#24121,#24122);
#20947=AXIS2_PLACEMENT_3D('',#60325,#24124,#24125);
#20948=AXIS2_PLACEMENT_3D('',#60326,#24126,#24127);
#20949=AXIS2_PLACEMENT_3D('',#60329,#24129,#24130);
#20950=AXIS2_PLACEMENT_3D('',#60330,#24131,#24132);
#20951=AXIS2_PLACEMENT_3D('',#60331,#24133,#24134);
#20952=AXIS2_PLACEMENT_3D('',#60333,#24135,#24136);
#20953=AXIS2_PLACEMENT_3D('',#60334,#24137,#24138);
#20954=AXIS2_PLACEMENT_3D('',#60335,#24139,#24140);
#20955=AXIS2_PLACEMENT_3D('',#60336,#24141,#24142);
#20956=AXIS2_PLACEMENT_3D('',#60340,#24144,#24145);
#20957=AXIS2_PLACEMENT_3D('',#60342,#24147,#24148);
#20958=AXIS2_PLACEMENT_3D('',#60346,#24151,#24152);
#20959=AXIS2_PLACEMENT_3D('',#60349,#24154,#24155);
#20960=AXIS2_PLACEMENT_3D('',#60350,#24156,#24157);
#20961=AXIS2_PLACEMENT_3D('',#60354,#24159,#24160);
#20962=AXIS2_PLACEMENT_3D('',#60356,#24162,#24163);
#20963=AXIS2_PLACEMENT_3D('',#60360,#24165,#24166);
#20964=AXIS2_PLACEMENT_3D('',#60362,#24168,#24169);
#20965=AXIS2_PLACEMENT_3D('',#60367,#24171,#24172);
#20966=AXIS2_PLACEMENT_3D('',#60370,#24174,#24175);
#20967=AXIS2_PLACEMENT_3D('',#60371,#24176,#24177);
#20968=AXIS2_PLACEMENT_3D('',#60374,#24179,#24180);
#20969=AXIS2_PLACEMENT_3D('',#60376,#24182,#24183);
#20970=AXIS2_PLACEMENT_3D('',#60377,#24184,#24185);
#20971=AXIS2_PLACEMENT_3D('',#60379,#24186,#24187);
#20972=AXIS2_PLACEMENT_3D('',#60380,#24188,#24189);
#20973=AXIS2_PLACEMENT_3D('',#60381,#24190,#24191);
#20974=AXIS2_PLACEMENT_3D('',#60382,#24192,#24193);
#20975=AXIS2_PLACEMENT_3D('',#60383,#24194,#24195);
#20976=AXIS2_PLACEMENT_3D('',#60385,#24197,#24198);
#20977=AXIS2_PLACEMENT_3D('',#60387,#24199,#24200);
#20978=AXIS2_PLACEMENT_3D('',#60389,#24201,#24202);
#20979=AXIS2_PLACEMENT_3D('',#60418,#24203,#24204);
#20980=AXIS2_PLACEMENT_3D('',#60421,#24207,#24208);
#20981=AXIS2_PLACEMENT_3D('',#60425,#24211,#24212);
#20982=AXIS2_PLACEMENT_3D('',#60429,#24215,#24216);
#20983=AXIS2_PLACEMENT_3D('',#60433,#24219,#24220);
#20984=AXIS2_PLACEMENT_3D('',#60436,#24222,#24223);
#20985=AXIS2_PLACEMENT_3D('',#60437,#24224,#24225);
#20986=AXIS2_PLACEMENT_3D('',#60441,#24228,#24229);
#20987=AXIS2_PLACEMENT_3D('',#60443,#24231,#24232);
#20988=AXIS2_PLACEMENT_3D('',#60445,#24234,#24235);
#20989=AXIS2_PLACEMENT_3D('',#60447,#24236,#24237);
#20990=AXIS2_PLACEMENT_3D('',#60449,#24239,#24240);
#20991=AXIS2_PLACEMENT_3D('',#60451,#24241,#24242);
#20992=AXIS2_PLACEMENT_3D('',#60453,#24243,#24244);
#20993=AXIS2_PLACEMENT_3D('',#60455,#24246,#24247);
#20994=AXIS2_PLACEMENT_3D('',#60457,#24248,#24249);
#20995=AXIS2_PLACEMENT_3D('',#60458,#24250,#24251);
#20996=AXIS2_PLACEMENT_3D('',#60459,#24252,#24253);
#20997=AXIS2_PLACEMENT_3D('',#60461,#24254,#24255);
#20998=AXIS2_PLACEMENT_3D('',#60463,#24257,#24258);
#20999=AXIS2_PLACEMENT_3D('',#60465,#24259,#24260);
#21000=AXIS2_PLACEMENT_3D('',#60467,#24261,#24262);
#21001=AXIS2_PLACEMENT_3D('',#60469,#24264,#24265);
#21002=AXIS2_PLACEMENT_3D('',#60474,#24267,#24268);
#21003=AXIS2_PLACEMENT_3D('',#60476,#24270,#24271);
#21004=AXIS2_PLACEMENT_3D('',#60477,#24272,#24273);
#21005=AXIS2_PLACEMENT_3D('',#60481,#24275,#24276);
#21006=AXIS2_PLACEMENT_3D('',#60482,#24277,#24278);
#21007=AXIS2_PLACEMENT_3D('',#60483,#24279,#24280);
#21008=AXIS2_PLACEMENT_3D('',#60485,#24282,#24283);
#21009=AXIS2_PLACEMENT_3D('',#60488,#24286,#24287);
#21010=AXIS2_PLACEMENT_3D('',#60490,#24289,#24290);
#21011=AXIS2_PLACEMENT_3D('',#60497,#24295,#24296);
#21012=AXIS2_PLACEMENT_3D('',#60500,#24297,#24298);
#21013=AXIS2_PLACEMENT_3D('',#60503,#24301,#24302);
#21014=AXIS2_PLACEMENT_3D('',#60505,#24303,#24304);
#21015=AXIS2_PLACEMENT_3D('',#60507,#24305,#24306);
#21016=AXIS2_PLACEMENT_3D('',#60536,#24307,#24308);
#21017=AXIS2_PLACEMENT_3D('',#60540,#24310,#24311);
#21018=AXIS2_PLACEMENT_3D('',#60542,#24313,#24314);
#21019=AXIS2_PLACEMENT_3D('',#60546,#24316,#24317);
#21020=AXIS2_PLACEMENT_3D('',#60548,#24319,#24320);
#21021=AXIS2_PLACEMENT_3D('',#60551,#24322,#24323);
#21022=AXIS2_PLACEMENT_3D('',#60552,#24324,#24325);
#21023=AXIS2_PLACEMENT_3D('',#60555,#24328,#24329);
#21024=AXIS2_PLACEMENT_3D('',#60559,#24332,#24333);
#21025=AXIS2_PLACEMENT_3D('',#60562,#24335,#24336);
#21026=AXIS2_PLACEMENT_3D('',#60563,#24337,#24338);
#21027=AXIS2_PLACEMENT_3D('',#60567,#24341,#24342);
#21028=AXIS2_PLACEMENT_3D('',#60571,#24345,#24346);
#21029=AXIS2_PLACEMENT_3D('',#60573,#24348,#24349);
#21030=AXIS2_PLACEMENT_3D('',#60576,#24351,#24352);
#21031=AXIS2_PLACEMENT_3D('',#60577,#24353,#24354);
#21032=AXIS2_PLACEMENT_3D('',#60579,#24355,#24356);
#21033=AXIS2_PLACEMENT_3D('',#60581,#24357,#24358);
#21034=AXIS2_PLACEMENT_3D('',#60610,#24359,#24360);
#21035=AXIS2_PLACEMENT_3D('',#60612,#24362,#24363);
#21036=AXIS2_PLACEMENT_3D('',#60615,#24365,#24366);
#21037=AXIS2_PLACEMENT_3D('',#60616,#24367,#24368);
#21038=AXIS2_PLACEMENT_3D('',#60619,#24370,#24371);
#21039=AXIS2_PLACEMENT_3D('',#60620,#24372,#24373);
#21040=AXIS2_PLACEMENT_3D('',#60622,#24375,#24376);
#21041=AXIS2_PLACEMENT_3D('',#60624,#24377,#24378);
#21042=AXIS2_PLACEMENT_3D('',#60626,#24379,#24380);
#21043=AXIS2_PLACEMENT_3D('',#60628,#24381,#24382);
#21044=AXIS2_PLACEMENT_3D('',#60629,#24383,#24384);
#21045=AXIS2_PLACEMENT_3D('',#60631,#24385,#24386);
#21046=AXIS2_PLACEMENT_3D('',#60633,#24387,#24388);
#21047=AXIS2_PLACEMENT_3D('',#60635,#24389,#24390);
#21048=AXIS2_PLACEMENT_3D('',#60636,#24391,#24392);
#21049=AXIS2_PLACEMENT_3D('',#60637,#24393,#24394);
#21050=AXIS2_PLACEMENT_3D('',#60639,#24395,#24396);
#21051=AXIS2_PLACEMENT_3D('',#60640,#24397,#24398);
#21052=AXIS2_PLACEMENT_3D('',#60643,#24400,#24401);
#21053=AXIS2_PLACEMENT_3D('',#60644,#24402,#24403);
#21054=AXIS2_PLACEMENT_3D('',#60646,#24404,#24405);
#21055=AXIS2_PLACEMENT_3D('',#60649,#24407,#24408);
#21056=AXIS2_PLACEMENT_3D('',#60650,#24409,#24410);
#21057=AXIS2_PLACEMENT_3D('',#60652,#24412,#24413);
#21058=AXIS2_PLACEMENT_3D('',#60655,#24415,#24416);
#21059=AXIS2_PLACEMENT_3D('',#60656,#24417,#24418);
#21060=AXIS2_PLACEMENT_3D('',#60659,#24420,#24421);
#21061=AXIS2_PLACEMENT_3D('',#60660,#24422,#24423);
#21062=AXIS2_PLACEMENT_3D('',#60663,#24425,#24426);
#21063=AXIS2_PLACEMENT_3D('',#60664,#24427,#24428);
#21064=AXIS2_PLACEMENT_3D('',#60695,#24430,#24431);
#21065=AXIS2_PLACEMENT_3D('',#60696,#24432,#24433);
#21066=AXIS2_PLACEMENT_3D('',#60697,#24434,#24435);
#21067=AXIS2_PLACEMENT_3D('',#60699,#24436,#24437);
#21068=AXIS2_PLACEMENT_3D('',#60701,#24438,#24439);
#21069=AXIS2_PLACEMENT_3D('',#60703,#24440,#24441);
#21070=AXIS2_PLACEMENT_3D('',#60704,#24442,#24443);
#21071=AXIS2_PLACEMENT_3D('',#60706,#24444,#24445);
#21072=AXIS2_PLACEMENT_3D('',#60708,#24446,#24447);
#21073=AXIS2_PLACEMENT_3D('',#60710,#24448,#24449);
#21074=AXIS2_PLACEMENT_3D('',#60711,#24450,#24451);
#21075=AXIS2_PLACEMENT_3D('',#60712,#24452,#24453);
#21076=AXIS2_PLACEMENT_3D('',#60714,#24454,#24455);
#21077=AXIS2_PLACEMENT_3D('',#60715,#24456,#24457);
#21078=AXIS2_PLACEMENT_3D('',#60718,#24459,#24460);
#21079=AXIS2_PLACEMENT_3D('',#60719,#24461,#24462);
#21080=AXIS2_PLACEMENT_3D('',#60721,#24463,#24464);
#21081=AXIS2_PLACEMENT_3D('',#60723,#24465,#24466);
#21082=AXIS2_PLACEMENT_3D('',#60724,#24467,#24468);
#21083=AXIS2_PLACEMENT_3D('',#60725,#24469,#24470);
#21084=AXIS2_PLACEMENT_3D('',#60729,#24472,#24473);
#21085=AXIS2_PLACEMENT_3D('',#60730,#24474,#24475);
#21086=AXIS2_PLACEMENT_3D('',#60731,#24476,#24477);
#21087=AXIS2_PLACEMENT_3D('',#60732,#24478,#24479);
#21088=AXIS2_PLACEMENT_3D('',#60733,#24480,#24481);
#21089=AXIS2_PLACEMENT_3D('',#60735,#24482,#24483);
#21090=AXIS2_PLACEMENT_3D('',#60737,#24484,#24485);
#21091=AXIS2_PLACEMENT_3D('',#60738,#24486,#24487);
#21092=AXIS2_PLACEMENT_3D('',#60739,#24488,#24489);
#21093=AXIS2_PLACEMENT_3D('',#60743,#24491,#24492);
#21094=AXIS2_PLACEMENT_3D('',#60744,#24493,#24494);
#21095=AXIS2_PLACEMENT_3D('',#60745,#24495,#24496);
#21096=AXIS2_PLACEMENT_3D('',#60746,#24497,#24498);
#21097=AXIS2_PLACEMENT_3D('',#60747,#24499,#24500);
#21098=AXIS2_PLACEMENT_3D('',#60749,#24501,#24502);
#21099=AXIS2_PLACEMENT_3D('',#60751,#24503,#24504);
#21100=AXIS2_PLACEMENT_3D('',#60752,#24505,#24506);
#21101=AXIS2_PLACEMENT_3D('',#60753,#24507,#24508);
#21102=AXIS2_PLACEMENT_3D('',#60756,#24509,#24510);
#21103=AXIS2_PLACEMENT_3D('',#60757,#24511,#24512);
#21104=AXIS2_PLACEMENT_3D('',#60759,#24514,#24515);
#21105=AXIS2_PLACEMENT_3D('',#60761,#24516,#24517);
#21106=AXIS2_PLACEMENT_3D('',#60762,#24518,#24519);
#21107=AXIS2_PLACEMENT_3D('',#60763,#24520,#24521);
#21108=AXIS2_PLACEMENT_3D('',#60765,#24522,#24523);
#21109=AXIS2_PLACEMENT_3D('',#60766,#24524,#24525);
#21110=AXIS2_PLACEMENT_3D('',#60768,#24526,#24527);
#21111=AXIS2_PLACEMENT_3D('',#60770,#24528,#24529);
#21112=AXIS2_PLACEMENT_3D('',#60771,#24530,#24531);
#21113=AXIS2_PLACEMENT_3D('',#60772,#24532,#24533);
#21114=AXIS2_PLACEMENT_3D('',#60775,#24534,#24535);
#21115=AXIS2_PLACEMENT_3D('',#60776,#24536,#24537);
#21116=AXIS2_PLACEMENT_3D('',#60778,#24539,#24540);
#21117=AXIS2_PLACEMENT_3D('',#60780,#24541,#24542);
#21118=AXIS2_PLACEMENT_3D('',#60781,#24543,#24544);
#21119=AXIS2_PLACEMENT_3D('',#60782,#24545,#24546);
#21120=AXIS2_PLACEMENT_3D('',#60785,#24548,#24549);
#21121=AXIS2_PLACEMENT_3D('',#60786,#24550,#24551);
#21122=AXIS2_PLACEMENT_3D('',#60788,#24552,#24553);
#21123=AXIS2_PLACEMENT_3D('',#60790,#24554,#24555);
#21124=AXIS2_PLACEMENT_3D('',#60791,#24556,#24557);
#21125=AXIS2_PLACEMENT_3D('',#60792,#24558,#24559);
#21126=AXIS2_PLACEMENT_3D('',#60795,#24560,#24561);
#21127=AXIS2_PLACEMENT_3D('',#60796,#24562,#24563);
#21128=AXIS2_PLACEMENT_3D('',#60798,#24565,#24566);
#21129=AXIS2_PLACEMENT_3D('',#60799,#24567,#24568);
#21130=AXIS2_PLACEMENT_3D('',#60800,#24569,#24570);
#21131=AXIS2_PLACEMENT_3D('',#60802,#24571,#24572);
#21132=AXIS2_PLACEMENT_3D('',#60804,#24573,#24574);
#21133=AXIS2_PLACEMENT_3D('',#60805,#24575,#24576);
#21134=AXIS2_PLACEMENT_3D('',#60806,#24577,#24578);
#21135=AXIS2_PLACEMENT_3D('',#60809,#24579,#24580);
#21136=AXIS2_PLACEMENT_3D('',#60810,#24581,#24582);
#21137=AXIS2_PLACEMENT_3D('',#60812,#24584,#24585);
#21138=AXIS2_PLACEMENT_3D('',#60813,#24586,#24587);
#21139=AXIS2_PLACEMENT_3D('',#60814,#24588,#24589);
#21140=AXIS2_PLACEMENT_3D('',#60816,#24590,#24591);
#21141=AXIS2_PLACEMENT_3D('',#60818,#24592,#24593);
#21142=AXIS2_PLACEMENT_3D('',#60820,#24594,#24595);
#21143=AXIS2_PLACEMENT_3D('',#60821,#24596,#24597);
#21144=AXIS2_PLACEMENT_3D('',#60822,#24598,#24599);
#21145=AXIS2_PLACEMENT_3D('',#60825,#24600,#24601);
#21146=AXIS2_PLACEMENT_3D('',#60826,#24602,#24603);
#21147=AXIS2_PLACEMENT_3D('',#60828,#24605,#24606);
#21148=AXIS2_PLACEMENT_3D('',#60838,#24612,#24613);
#21149=AXIS2_PLACEMENT_3D('',#60855,#24622,#24623);
#21150=AXIS2_PLACEMENT_3D('',#60858,#24625,#24626);
#21151=AXIS2_PLACEMENT_3D('',#60859,#24627,#24628);
#21152=AXIS2_PLACEMENT_3D('',#60860,#24629,#24630);
#21153=AXIS2_PLACEMENT_3D('',#60862,#24631,#24632);
#21154=AXIS2_PLACEMENT_3D('',#60864,#24634,#24635);
#21155=AXIS2_PLACEMENT_3D('',#60866,#24637,#24638);
#21156=AXIS2_PLACEMENT_3D('',#60870,#24641,#24642);
#21157=AXIS2_PLACEMENT_3D('',#60874,#24645,#24646);
#21158=AXIS2_PLACEMENT_3D('',#60876,#24648,#24649);
#21159=AXIS2_PLACEMENT_3D('',#60877,#24650,#24651);
#21160=AXIS2_PLACEMENT_3D('',#60879,#24652,#24653);
#21161=AXIS2_PLACEMENT_3D('',#60880,#24654,#24655);
#21162=AXIS2_PLACEMENT_3D('',#60881,#24656,#24657);
#21163=AXIS2_PLACEMENT_3D('',#60922,#24678,#24679);
#21164=AXIS2_PLACEMENT_3D('',#60923,#24680,#24681);
#21165=AXIS2_PLACEMENT_3D('',#60924,#24682,#24683);
#21166=AXIS2_PLACEMENT_3D('',#60925,#24684,#24685);
#21167=AXIS2_PLACEMENT_3D('',#60926,#24686,#24687);
#21168=AXIS2_PLACEMENT_3D('',#60927,#24688,#24689);
#21169=AXIS2_PLACEMENT_3D('',#60928,#24690,#24691);
#21170=AXIS2_PLACEMENT_3D('',#60929,#24692,#24693);
#21171=AXIS2_PLACEMENT_3D('',#60930,#24694,#24695);
#21172=AXIS2_PLACEMENT_3D('',#60932,#24696,#24697);
#21173=AXIS2_PLACEMENT_3D('',#60934,#24698,#24699);
#21174=AXIS2_PLACEMENT_3D('',#60935,#24700,#24701);
#21175=AXIS2_PLACEMENT_3D('',#60936,#24702,#24703);
#21176=AXIS2_PLACEMENT_3D('',#60940,#24705,#24706);
#21177=AXIS2_PLACEMENT_3D('',#60941,#24707,#24708);
#21178=AXIS2_PLACEMENT_3D('',#60942,#24709,#24710);
#21179=AXIS2_PLACEMENT_3D('',#60943,#24711,#24712);
#21180=AXIS2_PLACEMENT_3D('',#60944,#24713,#24714);
#21181=AXIS2_PLACEMENT_3D('',#60946,#24715,#24716);
#21182=AXIS2_PLACEMENT_3D('',#60949,#24718,#24719);
#21183=AXIS2_PLACEMENT_3D('',#60950,#24720,#24721);
#21184=AXIS2_PLACEMENT_3D('',#60953,#24723,#24724);
#21185=AXIS2_PLACEMENT_3D('',#60954,#24725,#24726);
#21186=AXIS2_PLACEMENT_3D('',#60957,#24728,#24729);
#21187=AXIS2_PLACEMENT_3D('',#60958,#24730,#24731);
#21188=AXIS2_PLACEMENT_3D('',#60960,#24733,#24734);
#21189=AXIS2_PLACEMENT_3D('',#60966,#24738,#24739);
#21190=AXIS2_PLACEMENT_3D('',#60970,#24742,#24743);
#21191=AXIS2_PLACEMENT_3D('',#60971,#24744,#24745);
#21192=AXIS2_PLACEMENT_3D('',#60972,#24746,#24747);
#21193=AXIS2_PLACEMENT_3D('',#60973,#24748,#24749);
#21194=AXIS2_PLACEMENT_3D('',#60974,#24750,#24751);
#21195=AXIS2_PLACEMENT_3D('',#60975,#24752,#24753);
#21196=AXIS2_PLACEMENT_3D('',#60977,#24754,#24755);
#21197=AXIS2_PLACEMENT_3D('',#60979,#24757,#24758);
#21198=AXIS2_PLACEMENT_3D('',#60981,#24760,#24761);
#21199=AXIS2_PLACEMENT_3D('',#60983,#24762,#24763);
#21200=AXIS2_PLACEMENT_3D('',#60986,#24765,#24766);
#21201=AXIS2_PLACEMENT_3D('',#60987,#24767,#24768);
#21202=AXIS2_PLACEMENT_3D('',#60990,#24770,#24771);
#21203=AXIS2_PLACEMENT_3D('',#60991,#24772,#24773);
#21204=AXIS2_PLACEMENT_3D('',#60994,#24775,#24776);
#21205=AXIS2_PLACEMENT_3D('',#60995,#24777,#24778);
#21206=AXIS2_PLACEMENT_3D('',#60997,#24780,#24781);
#21207=AXIS2_PLACEMENT_3D('',#61003,#24785,#24786);
#21208=AXIS2_PLACEMENT_3D('',#61007,#24789,#24790);
#21209=AXIS2_PLACEMENT_3D('',#61008,#24791,#24792);
#21210=AXIS2_PLACEMENT_3D('',#61009,#24793,#24794);
#21211=AXIS2_PLACEMENT_3D('',#61010,#24795,#24796);
#21212=AXIS2_PLACEMENT_3D('',#61011,#24797,#24798);
#21213=AXIS2_PLACEMENT_3D('',#61012,#24799,#24800);
#21214=AXIS2_PLACEMENT_3D('',#61014,#24801,#24802);
#21215=AXIS2_PLACEMENT_3D('',#61016,#24804,#24805);
#21216=AXIS2_PLACEMENT_3D('',#61018,#24807,#24808);
#21217=AXIS2_PLACEMENT_3D('',#61021,#24809,#24810);
#21218=AXIS2_PLACEMENT_3D('',#61025,#24812,#24813);
#21219=AXIS2_PLACEMENT_3D('',#61029,#24815,#24816);
#21220=AXIS2_PLACEMENT_3D('',#61031,#24818,#24819);
#21221=AXIS2_PLACEMENT_3D('',#61033,#24820,#24821);
#21222=AXIS2_PLACEMENT_3D('',#61036,#24823,#24824);
#21223=AXIS2_PLACEMENT_3D('',#61037,#24825,#24826);
#21224=AXIS2_PLACEMENT_3D('',#61041,#24828,#24829);
#21225=AXIS2_PLACEMENT_3D('',#61043,#24830,#24831);
#21226=AXIS2_PLACEMENT_3D('',#61046,#24834,#24835);
#21227=AXIS2_PLACEMENT_3D('',#61048,#24837,#24838);
#21228=AXIS2_PLACEMENT_3D('',#61052,#24840,#24841);
#21229=AXIS2_PLACEMENT_3D('',#61054,#24842,#24843);
#21230=AXIS2_PLACEMENT_3D('',#61056,#24845,#24846);
#21231=AXIS2_PLACEMENT_3D('',#61059,#24847,#24848);
#21232=AXIS2_PLACEMENT_3D('',#61063,#24852,#24853);
#21233=AXIS2_PLACEMENT_3D('',#61065,#24855,#24856);
#21234=AXIS2_PLACEMENT_3D('',#61067,#24858,#24859);
#21235=AXIS2_PLACEMENT_3D('',#61068,#24860,#24861);
#21236=AXIS2_PLACEMENT_3D('',#61070,#24863,#24864);
#21237=AXIS2_PLACEMENT_3D('',#61073,#24865,#24866);
#21238=AXIS2_PLACEMENT_3D('',#61077,#24868,#24869);
#21239=AXIS2_PLACEMENT_3D('',#61081,#24871,#24872);
#21240=AXIS2_PLACEMENT_3D('',#61083,#24874,#24875);
#21241=AXIS2_PLACEMENT_3D('',#61085,#24876,#24877);
#21242=AXIS2_PLACEMENT_3D('',#61088,#24879,#24880);
#21243=AXIS2_PLACEMENT_3D('',#61089,#24881,#24882);
#21244=AXIS2_PLACEMENT_3D('',#61093,#24884,#24885);
#21245=AXIS2_PLACEMENT_3D('',#61095,#24886,#24887);
#21246=AXIS2_PLACEMENT_3D('',#61098,#24890,#24891);
#21247=AXIS2_PLACEMENT_3D('',#61100,#24893,#24894);
#21248=AXIS2_PLACEMENT_3D('',#61104,#24896,#24897);
#21249=AXIS2_PLACEMENT_3D('',#61106,#24898,#24899);
#21250=AXIS2_PLACEMENT_3D('',#61108,#24901,#24902);
#21251=AXIS2_PLACEMENT_3D('',#61111,#24903,#24904);
#21252=AXIS2_PLACEMENT_3D('',#61115,#24908,#24909);
#21253=AXIS2_PLACEMENT_3D('',#61117,#24911,#24912);
#21254=AXIS2_PLACEMENT_3D('',#61119,#24914,#24915);
#21255=AXIS2_PLACEMENT_3D('',#61120,#24916,#24917);
#21256=AXIS2_PLACEMENT_3D('',#61122,#24919,#24920);
#21257=AXIS2_PLACEMENT_3D('',#61123,#24921,#24922);
#21258=AXIS2_PLACEMENT_3D('',#61124,#24923,#24924);
#21259=AXIS2_PLACEMENT_3D('',#61125,#24925,#24926);
#21260=AXIS2_PLACEMENT_3D('',#61126,#24927,#24928);
#23945=DIRECTION('axis',(0.,0.,1.));
#23946=DIRECTION('refdir',(1.,0.,0.));
#23947=DIRECTION('center_axis',(0.,1.,0.));
#23948=DIRECTION('ref_axis',(-0.707106781186548,0.,0.707106781186548));
#23949=DIRECTION('',(0.,-1.,0.));
#23950=DIRECTION('center_axis',(0.,0.707106781186548,-0.707106781186548));
#23951=DIRECTION('ref_axis',(0.,-0.707106781186548,-0.707106781186548));
#23952=DIRECTION('',(0.,1.,0.));
#23953=DIRECTION('center_axis',(0.,-0.707106781186548,-0.707106781186548));
#23954=DIRECTION('ref_axis',(0.,-0.707106781186548,0.707106781186548));
#23955=DIRECTION('center_axis',(0.,0.,-1.));
#23956=DIRECTION('ref_axis',(-0.707106781186548,0.707106781186548,0.));
#23957=DIRECTION('',(0.,0.,-1.));
#23958=DIRECTION('',(0.,0.,1.));
#23959=DIRECTION('center_axis',(0.,0.707106781186548,0.707106781186548));
#23960=DIRECTION('ref_axis',(0.,0.707106781186548,-0.707106781186548));
#23961=DIRECTION('center_axis',(0.,0.,1.));
#23962=DIRECTION('ref_axis',(-0.707106781186548,-0.707106781186548,0.));
#23963=DIRECTION('',(0.,0.,-1.));
#23964=DIRECTION('',(0.,0.,1.));
#23965=DIRECTION('center_axis',(0.,0.707106781186548,-0.707106781186548));
#23966=DIRECTION('ref_axis',(0.,-0.707106781186548,-0.707106781186548));
#23967=DIRECTION('center_axis',(0.,-1.,0.));
#23968=DIRECTION('ref_axis',(-0.70710678118654,0.,-0.707106781186555));
#23969=DIRECTION('',(0.,1.,0.));
#23970=DIRECTION('',(0.,-1.,0.));
#23971=DIRECTION('center_axis',(0.,1.,0.));
#23972=DIRECTION('ref_axis',(0.,0.,-1.));
#23973=DIRECTION('',(-1.,0.,0.));
#23974=DIRECTION('',(0.,0.,-1.));
#23975=DIRECTION('',(-1.,0.,0.));
#23976=DIRECTION('center_axis',(0.,0.,-1.));
#23977=DIRECTION('ref_axis',(0.,-1.,0.));
#23978=DIRECTION('',(-1.,0.,0.));
#23979=DIRECTION('',(0.,-1.,0.));
#23980=DIRECTION('center_axis',(-1.,0.,0.));
#23981=DIRECTION('ref_axis',(0.,0.,1.));
#23982=DIRECTION('',(0.,0.985211754819674,-0.171341174751248));
#23983=DIRECTION('center_axis',(1.,0.,0.));
#23984=DIRECTION('ref_axis',(0.,6.13317366673349E-17,-1.));
#23985=DIRECTION('',(0.,1.,0.));
#23986=DIRECTION('',(0.,0.,-1.));
#23987=DIRECTION('',(0.,-1.,0.));
#23988=DIRECTION('',(0.,0.,-1.));
#23989=DIRECTION('center_axis',(0.,0.985211754819675,-0.171341174751248));
#23990=DIRECTION('ref_axis',(-0.707106781186549,-0.121156506563076,-0.696649912737688));
#23991=DIRECTION('center_axis',(0.,1.,0.));
#23992=DIRECTION('ref_axis',(2.13633744986749E-15,0.,-1.));
#23993=DIRECTION('',(0.,-0.985211754819674,0.171341174751248));
#23994=DIRECTION('center_axis',(0.,1.,0.));
#23995=DIRECTION('ref_axis',(0.70710678118654,0.,-0.707106781186555));
#23996=DIRECTION('',(0.,-1.,0.));
#23997=DIRECTION('center_axis',(0.,0.707106781186548,0.707106781186548));
#23998=DIRECTION('ref_axis',(0.,-0.707106781186548,0.707106781186548));
#23999=DIRECTION('',(0.,1.,0.));
#24000=DIRECTION('center_axis',(0.,0.707106781186548,-0.707106781186548));
#24001=DIRECTION('ref_axis',(0.,0.707106781186548,0.707106781186548));
#24002=DIRECTION('center_axis',(0.,-1.,0.));
#24003=DIRECTION('ref_axis',(0.707106781186548,0.,0.707106781186548));
#24004=DIRECTION('',(0.,1.,0.));
#24005=DIRECTION('center_axis',(0.,-0.707106781186548,-0.707106781186548));
#24006=DIRECTION('ref_axis',(0.,0.707106781186548,-0.707106781186548));
#24007=DIRECTION('center_axis',(0.,0.707106781186548,-0.707106781186548));
#24008=DIRECTION('ref_axis',(0.,0.707106781186548,0.707106781186548));
#24009=DIRECTION('center_axis',(0.,0.,-1.));
#24010=DIRECTION('ref_axis',(0.707106781186548,-0.707106781186548,0.));
#24011=DIRECTION('',(0.,0.,1.));
#24012=DIRECTION('center_axis',(0.,0.,1.));
#24013=DIRECTION('ref_axis',(0.707106781186548,0.707106781186548,0.));
#24014=DIRECTION('',(0.,0.,-1.));
#24015=DIRECTION('',(0.,0.,1.));
#24016=DIRECTION('center_axis',(0.,-1.,0.));
#24017=DIRECTION('ref_axis',(0.,0.,1.));
#24018=DIRECTION('',(-1.,0.,0.));
#24019=DIRECTION('center_axis',(1.,0.,0.));
#24020=DIRECTION('ref_axis',(0.,0.,-1.));
#24021=DIRECTION('',(0.,-0.985211754819674,0.171341174751248));
#24022=DIRECTION('',(0.,0.,1.));
#24023=DIRECTION('',(0.,1.,0.));
#24024=DIRECTION('',(0.,0.,-1.));
#24025=DIRECTION('',(0.,1.,0.));
#24026=DIRECTION('',(0.,0.,1.));
#24027=DIRECTION('center_axis',(0.,0.985211754819675,-0.171341174751248));
#24028=DIRECTION('ref_axis',(0.707106781186549,-0.121156506563076,-0.696649912737688));
#24029=DIRECTION('center_axis',(0.,0.64368424916598,-0.76529117816399));
#24030=DIRECTION('ref_axis',(-1.99135285907852E-16,-0.76529117816399,-0.64368424916598));
#24031=DIRECTION('center_axis',(0.,-1.,0.));
#24032=DIRECTION('ref_axis',(-2.13633744986749E-15,0.,-1.));
#24033=DIRECTION('',(0.,0.985211754819674,-0.171341174751248));
#24034=DIRECTION('center_axis',(0.,-0.985211754819675,0.171341174751248));
#24035=DIRECTION('ref_axis',(0.707106781186549,-0.121156506563076,-0.696649912737688));
#24036=DIRECTION('',(0.,0.985211754819674,-0.171341174751248));
#24037=DIRECTION('center_axis',(0.,1.,0.));
#24038=DIRECTION('ref_axis',(-1.96543045387809E-15,0.,-1.));
#24039=DIRECTION('',(0.,-0.985211754819674,0.171341174751248));
#24040=DIRECTION('center_axis',(0.,-0.171341174751248,-0.985211754819675));
#24041=DIRECTION('ref_axis',(0.,0.985211754819675,-0.171341174751248));
#24042=DIRECTION('center_axis',(0.,0.171341174751248,0.985211754819675));
#24043=DIRECTION('ref_axis',(0.985636596769451,-0.166382691564751,0.0289361202721306));
#24044=DIRECTION('',(1.,0.,0.));
#24045=DIRECTION('',(0.,-0.985211754819674,0.171341174751248));
#24046=DIRECTION('',(1.,0.,0.));
#24047=DIRECTION('center_axis',(0.,1.,0.));
#24048=DIRECTION('ref_axis',(0.70710678118654,0.,-0.707106781186555));
#24049=DIRECTION('',(0.,-1.,0.));
#24050=DIRECTION('center_axis',(0.,0.707106781186548,0.707106781186548));
#24051=DIRECTION('ref_axis',(0.,-0.707106781186548,0.707106781186548));
#24052=DIRECTION('',(0.,1.,0.));
#24053=DIRECTION('center_axis',(0.,-0.707106781186548,0.707106781186548));
#24054=DIRECTION('ref_axis',(0.,-0.707106781186548,-0.707106781186548));
#24055=DIRECTION('center_axis',(0.,0.,1.));
#24056=DIRECTION('ref_axis',(0.707106781186548,0.707106781186548,0.));
#24057=DIRECTION('',(0.,0.,1.));
#24058=DIRECTION('',(0.,0.,-1.));
#24059=DIRECTION('center_axis',(0.,0.707106781186548,-0.707106781186548));
#24060=DIRECTION('ref_axis',(0.,0.707106781186548,0.707106781186548));
#24061=DIRECTION('center_axis',(0.,0.,-1.));
#24062=DIRECTION('ref_axis',(0.707106781186548,-0.707106781186548,0.));
#24063=DIRECTION('',(0.,0.,1.));
#24064=DIRECTION('',(0.,0.,-1.));
#24065=DIRECTION('center_axis',(0.,0.707106781186548,0.707106781186548));
#24066=DIRECTION('ref_axis',(0.,-0.707106781186548,0.707106781186548));
#24067=DIRECTION('center_axis',(0.,-1.,0.));
#24068=DIRECTION('ref_axis',(0.707106781186548,0.,0.707106781186548));
#24069=DIRECTION('',(0.,1.,0.));
#24070=DIRECTION('',(0.,-1.,0.));
#24071=DIRECTION('center_axis',(0.,1.,0.));
#24072=DIRECTION('ref_axis',(0.,0.,1.));
#24073=DIRECTION('',(1.,0.,0.));
#24074=DIRECTION('',(0.,0.,1.));
#24075=DIRECTION('',(1.,0.,0.));
#24076=DIRECTION('center_axis',(0.,0.,1.));
#24077=DIRECTION('ref_axis',(0.,-1.,0.));
#24078=DIRECTION('',(1.,0.,0.));
#24079=DIRECTION('',(0.,-1.,0.));
#24080=DIRECTION('center_axis',(1.,0.,0.));
#24081=DIRECTION('ref_axis',(0.,0.,-1.));
#24082=DIRECTION('',(0.,0.,1.));
#24083=DIRECTION('',(0.,1.,0.));
#24084=DIRECTION('',(0.,0.,1.));
#24085=DIRECTION('',(0.,1.,0.));
#24086=DIRECTION('center_axis',(-1.,0.,0.));
#24087=DIRECTION('ref_axis',(0.,6.13317366673349E-17,-1.));
#24088=DIRECTION('center_axis',(0.40824829046386,-0.816496580927729,0.40824829046386));
#24089=DIRECTION('ref_axis',(0.577350269189632,0.577350269189623,0.577350269189623));
#24090=DIRECTION('center_axis',(0.,1.,0.));
#24091=DIRECTION('ref_axis',(0.,0.,1.));
#24092=DIRECTION('center_axis',(0.,0.,1.));
#24093=DIRECTION('ref_axis',(0.707106781186545,0.70710678118655,0.));
#24094=DIRECTION('center_axis',(1.,0.,0.));
#24095=DIRECTION('ref_axis',(0.,0.707106781186542,0.707106781186553));
#24096=DIRECTION('center_axis',(0.,-1.,0.));
#24097=DIRECTION('ref_axis',(0.70710678118654,0.,0.707106781186555));
#24098=DIRECTION('center_axis',(0.707106781186548,-0.707106781186548,0.));
#24099=DIRECTION('ref_axis',(0.707106781186548,0.707106781186548,0.));
#24100=DIRECTION('',(0.,-1.,0.));
#24101=DIRECTION('center_axis',(0.,0.,1.));
#24102=DIRECTION('ref_axis',(1.,0.,0.));
#24103=DIRECTION('',(1.,0.,0.));
#24104=DIRECTION('',(1.,0.,0.));
#24105=DIRECTION('',(0.,1.,0.));
#24106=DIRECTION('',(-1.,0.,0.));
#24107=DIRECTION('',(0.,1.,0.));
#24108=DIRECTION('',(-1.,0.,0.));
#24109=DIRECTION('',(0.,-1.,0.));
#24110=DIRECTION('',(-1.,0.,0.));
#24111=DIRECTION('',(0.,1.,0.));
#24112=DIRECTION('',(1.,0.,0.));
#24113=DIRECTION('',(0.,1.,0.));
#24114=DIRECTION('center_axis',(1.,0.,0.));
#24115=DIRECTION('ref_axis',(0.,0.70710678118654,0.707106781186555));
#24116=DIRECTION('',(-1.,0.,0.));
#24117=DIRECTION('center_axis',(0.987087457637498,0.,0.160182243006963));
#24118=DIRECTION('ref_axis',(-0.160182243006963,0.,0.987087457637497));
#24119=DIRECTION('center_axis',(0.,0.,-1.));
#24120=DIRECTION('ref_axis',(0.707106781186548,0.707106781186548,0.));
#24121=DIRECTION('center_axis',(-0.707106781186548,0.,-0.707106781186548));
#24122=DIRECTION('ref_axis',(0.707106781186548,0.,-0.707106781186548));
#24123=DIRECTION('',(0.,0.,1.));
#24124=DIRECTION('center_axis',(1.,0.,0.));
#24125=DIRECTION('ref_axis',(0.,-0.70710678118654,0.707106781186555));
#24126=DIRECTION('center_axis',(0.707106781186546,0.707106781186549,0.));
#24127=DIRECTION('ref_axis',(-0.707106781186549,0.707106781186546,0.));
#24128=DIRECTION('',(1.,0.,0.));
#24129=DIRECTION('center_axis',(-0.987087457637496,-2.19177444557571E-14,
0.160182243006974));
#24130=DIRECTION('ref_axis',(-0.160182243006974,1.35063227020986E-13,-0.987087457637496));
#24131=DIRECTION('center_axis',(-0.408248290463859,-0.81649658092773,-0.408248290463859));
#24132=DIRECTION('ref_axis',(0.577350269189621,-0.577350269189618,0.577350269189638));
#24133=DIRECTION('center_axis',(0.,-1.,0.));
#24134=DIRECTION('ref_axis',(1.,0.,0.));
#24135=DIRECTION('center_axis',(1.,0.,0.));
#24136=DIRECTION('ref_axis',(0.,-0.707106781186542,0.707106781186553));
#24137=DIRECTION('center_axis',(0.,0.,1.));
#24138=DIRECTION('ref_axis',(0.707106781186549,-0.707106781186546,0.));
#24139=DIRECTION('center_axis',(0.,1.,0.));
#24140=DIRECTION('ref_axis',(0.707106781186555,0.,0.70710678118654));
#24141=DIRECTION('center_axis',(0.948683298050514,0.,-0.316227766016838));
#24142=DIRECTION('ref_axis',(0.223606797749977,-0.707106781186554,0.670820393249931));
#24143=DIRECTION('',(0.948683298050514,0.,-0.316227766016838));
#24144=DIRECTION('center_axis',(0.987087457637496,0.,-0.160182243006974));
#24145=DIRECTION('ref_axis',(0.160182243006974,3.42464757121206E-15,0.987087457637496));
#24146=DIRECTION('',(-0.948683298050514,0.,0.316227766016838));
#24147=DIRECTION('center_axis',(0.316227766016838,0.,0.948683298050514));
#24148=DIRECTION('ref_axis',(0.948683298050514,0.,-0.316227766016838));
#24149=DIRECTION('',(0.,1.,0.));
#24150=DIRECTION('',(0.948683298050514,0.,-0.316227766016838));
#24151=DIRECTION('center_axis',(0.,0.,1.));
#24152=DIRECTION('ref_axis',(0.707106781186548,-0.707106781186548,0.));
#24153=DIRECTION('',(0.,0.,-1.));
#24154=DIRECTION('center_axis',(0.707106781186548,0.,0.707106781186548));
#24155=DIRECTION('ref_axis',(0.707106781186548,0.,-0.707106781186548));
#24156=DIRECTION('center_axis',(1.,0.,0.));
#24157=DIRECTION('ref_axis',(0.,-0.707106781186548,-0.707106781186548));
#24158=DIRECTION('',(-1.,0.,0.));
#24159=DIRECTION('center_axis',(0.988554494713122,0.,-0.150864213723747));
#24160=DIRECTION('ref_axis',(-0.150864213723747,0.,-0.988554494713122));
#24161=DIRECTION('',(1.,0.,0.));
#24162=DIRECTION('center_axis',(0.95447997803503,0.,-0.298274993135947));
#24163=DIRECTION('ref_axis',(-0.210912270304798,-0.707106781186552,-0.674919264975352));
#24164=DIRECTION('',(-0.95447997803503,0.,0.298274993135947));
#24165=DIRECTION('center_axis',(0.855572029308621,0.,-0.517683786364541));
#24166=DIRECTION('ref_axis',(-0.517683786364541,0.,-0.855572029308621));
#24167=DIRECTION('',(0.95447997803503,0.,-0.298274993135947));
#24168=DIRECTION('center_axis',(-1.,0.,0.));
#24169=DIRECTION('ref_axis',(0.,-0.70710678118654,0.707106781186555));
#24170=DIRECTION('',(-1.,0.,0.));
#24171=DIRECTION('center_axis',(1.,0.,0.));
#24172=DIRECTION('ref_axis',(0.,0.,1.));
#24173=DIRECTION('',(1.,0.,0.));
#24174=DIRECTION('center_axis',(-0.987087457637498,0.,-0.160182243006963));
#24175=DIRECTION('ref_axis',(0.160182243006963,0.,-0.987087457637497));
#24176=DIRECTION('center_axis',(-0.948683298050514,0.,-0.316227766016838));
#24177=DIRECTION('ref_axis',(-0.223606797749977,-0.707106781186554,0.670820393249931));
#24178=DIRECTION('',(0.948683298050514,0.,0.316227766016838));
#24179=DIRECTION('center_axis',(-0.987087457637498,0.,-0.160182243006963));
#24180=DIRECTION('ref_axis',(-0.160182243006963,0.,0.987087457637497));
#24181=DIRECTION('',(-0.948683298050514,0.,-0.316227766016838));
#24182=DIRECTION('center_axis',(0.40824829046386,-0.81649658092773,-0.40824829046386));
#24183=DIRECTION('ref_axis',(-0.57735026918962,-0.577350269189619,0.577350269189638));
#24184=DIRECTION('center_axis',(0.,-1.,0.));
#24185=DIRECTION('ref_axis',(0.,0.,1.));
#24186=DIRECTION('center_axis',(0.,0.,1.));
#24187=DIRECTION('ref_axis',(-0.707106781186549,-0.707106781186546,0.));
#24188=DIRECTION('center_axis',(-1.,0.,0.));
#24189=DIRECTION('ref_axis',(0.,-0.707106781186542,0.707106781186553));
#24190=DIRECTION('center_axis',(0.,1.,0.));
#24191=DIRECTION('ref_axis',(-0.70710678118654,0.,0.707106781186555));
#24192=DIRECTION('center_axis',(0.707106781186546,-0.707106781186549,0.));
#24193=DIRECTION('ref_axis',(-0.707106781186549,-0.707106781186546,0.));
#24194=DIRECTION('center_axis',(-1.,0.,0.));
#24195=DIRECTION('ref_axis',(0.,-0.70710678118654,0.707106781186555));
#24196=DIRECTION('',(1.,0.,0.));
#24197=DIRECTION('center_axis',(0.,1.,0.));
#24198=DIRECTION('ref_axis',(-0.999898028249439,0.,-0.0142805147975766));
#24199=DIRECTION('center_axis',(0.,1.,0.));
#24200=DIRECTION('ref_axis',(-1.,0.,0.));
#24201=DIRECTION('center_axis',(0.,-1.,0.));
#24202=DIRECTION('ref_axis',(-1.,0.,0.));
#24203=DIRECTION('center_axis',(0.707106781186548,0.,-0.707106781186548));
#24204=DIRECTION('ref_axis',(-0.500000000000001,-0.707106781186546,-0.500000000000001));
#24205=DIRECTION('',(-0.707106781186547,0.,0.707106781186547));
#24206=DIRECTION('',(0.707106781186547,0.,-0.707106781186547));
#24207=DIRECTION('center_axis',(0.,0.,-1.));
#24208=DIRECTION('ref_axis',(-1.,0.,0.));
#24209=DIRECTION('',(0.,1.,0.));
#24210=DIRECTION('',(-1.,0.,0.));
#24211=DIRECTION('center_axis',(-0.298274993135947,0.,-0.95447997803503));
#24212=DIRECTION('ref_axis',(-0.95447997803503,0.,0.298274993135947));
#24213=DIRECTION('',(0.,1.,0.));
#24214=DIRECTION('',(-0.95447997803503,0.,0.298274993135947));
#24215=DIRECTION('center_axis',(-0.707106781186548,0.,-0.707106781186548));
#24216=DIRECTION('ref_axis',(-0.707106781186548,0.,0.707106781186548));
#24217=DIRECTION('',(0.,1.,0.));
#24218=DIRECTION('',(-0.707106781186547,0.,0.707106781186547));
#24219=DIRECTION('center_axis',(0.,1.,0.));
#24220=DIRECTION('ref_axis',(0.,0.,-1.));
#24221=DIRECTION('',(0.,1.,0.));
#24222=DIRECTION('center_axis',(0.,1.,0.));
#24223=DIRECTION('ref_axis',(-1.,0.,0.));
#24224=DIRECTION('center_axis',(0.,0.,1.));
#24225=DIRECTION('ref_axis',(1.,0.,0.));
#24226=DIRECTION('',(0.,1.,0.));
#24227=DIRECTION('',(1.,0.,0.));
#24228=DIRECTION('center_axis',(-0.316227766016838,0.,0.948683298050514));
#24229=DIRECTION('ref_axis',(0.948683298050514,0.,0.316227766016838));
#24230=DIRECTION('',(0.948683298050514,0.,0.316227766016838));
#24231=DIRECTION('center_axis',(1.,0.,0.));
#24232=DIRECTION('ref_axis',(0.,-0.707106781186539,0.707106781186556));
#24233=DIRECTION('',(1.,0.,0.));
#24234=DIRECTION('center_axis',(0.,0.,1.));
#24235=DIRECTION('ref_axis',(-0.707106781186548,-0.707106781186547,0.));
#24236=DIRECTION('center_axis',(-0.382683432365102,0.,0.923879532511282));
#24237=DIRECTION('ref_axis',(-0.923879532511282,0.,-0.382683432365102));
#24238=DIRECTION('',(0.,0.,1.));
#24239=DIRECTION('center_axis',(0.,1.,0.));
#24240=DIRECTION('ref_axis',(-0.70710678118654,0.,0.707106781186555));
#24241=DIRECTION('center_axis',(-0.707106781186547,-0.707106781186548,0.));
#24242=DIRECTION('ref_axis',(-0.707106781186548,0.707106781186547,0.));
#24243=DIRECTION('center_axis',(0.,-1.,0.));
#24244=DIRECTION('ref_axis',(0.,0.,1.));
#24245=DIRECTION('',(0.,-1.,0.));
#24246=DIRECTION('center_axis',(-0.40824829046386,-0.816496580927729,0.40824829046386));
#24247=DIRECTION('ref_axis',(-0.577350269189632,0.577350269189623,0.577350269189623));
#24248=DIRECTION('center_axis',(-1.,0.,0.));
#24249=DIRECTION('ref_axis',(0.,0.707106781186542,0.707106781186553));
#24250=DIRECTION('center_axis',(0.,0.,1.));
#24251=DIRECTION('ref_axis',(-0.707106781186545,0.70710678118655,0.));
#24252=DIRECTION('center_axis',(1.,0.,0.));
#24253=DIRECTION('ref_axis',(0.,0.70710678118654,0.707106781186555));
#24254=DIRECTION('center_axis',(0.987087457637498,-1.09588722278786E-14,
-0.160182243006963));
#24255=DIRECTION('ref_axis',(0.160182243006963,-6.7531613510494E-14,0.987087457637497));
#24256=DIRECTION('',(-1.,0.,0.));
#24257=DIRECTION('center_axis',(0.,0.985211754819675,-0.171341174751248));
#24258=DIRECTION('ref_axis',(-0.707106781186549,-0.121156506563076,-0.696649912737688));
#24259=DIRECTION('center_axis',(0.,0.64368424916598,-0.76529117816399));
#24260=DIRECTION('ref_axis',(1.99135285907852E-16,-0.76529117816399,-0.64368424916598));
#24261=DIRECTION('center_axis',(0.,-1.,0.));
#24262=DIRECTION('ref_axis',(2.13633744986749E-15,0.,-1.));
#24263=DIRECTION('',(0.,0.985211754819674,-0.171341174751248));
#24264=DIRECTION('center_axis',(0.,1.,0.));
#24265=DIRECTION('ref_axis',(-0.707106781186548,0.,0.707106781186548));
#24266=DIRECTION('',(0.,-1.,0.));
#24267=DIRECTION('center_axis',(0.,0.707106781186548,-0.707106781186548));
#24268=DIRECTION('ref_axis',(0.,-0.707106781186548,-0.707106781186548));
#24269=DIRECTION('',(0.,1.,0.));
#24270=DIRECTION('center_axis',(0.,0.707106781186548,0.707106781186548));
#24271=DIRECTION('ref_axis',(0.,0.707106781186548,-0.707106781186548));
#24272=DIRECTION('center_axis',(0.,-1.,0.));
#24273=DIRECTION('ref_axis',(-0.70710678118654,0.,-0.707106781186555));
#24274=DIRECTION('',(0.,1.,0.));
#24275=DIRECTION('center_axis',(0.,-0.707106781186548,0.707106781186548));
#24276=DIRECTION('ref_axis',(0.,0.707106781186548,0.707106781186548));
#24277=DIRECTION('center_axis',(0.,0.707106781186548,0.707106781186548));
#24278=DIRECTION('ref_axis',(0.,0.707106781186548,-0.707106781186548));
#24279=DIRECTION('center_axis',(0.,0.,1.));
#24280=DIRECTION('ref_axis',(-0.707106781186548,-0.707106781186548,0.));
#24281=DIRECTION('',(0.,0.,-1.));
#24282=DIRECTION('center_axis',(0.,0.,-1.));
#24283=DIRECTION('ref_axis',(-0.707106781186548,0.707106781186548,0.));
#24284=DIRECTION('',(0.,0.,1.));
#24285=DIRECTION('',(0.,0.,-1.));
#24286=DIRECTION('center_axis',(0.,-1.,0.));
#24287=DIRECTION('ref_axis',(0.,0.,-1.));
#24288=DIRECTION('',(1.,0.,0.));
#24289=DIRECTION('center_axis',(1.,0.,0.));
#24290=DIRECTION('ref_axis',(0.,0.,-1.));
#24291=DIRECTION('',(0.,0.,1.));
#24292=DIRECTION('',(0.,1.,0.));
#24293=DIRECTION('',(0.,0.,-1.));
#24294=DIRECTION('',(0.,0.,-1.));
#24295=DIRECTION('center_axis',(1.,0.,0.));
#24296=DIRECTION('ref_axis',(0.,-0.70710678118654,0.707106781186555));
#24297=DIRECTION('center_axis',(-1.,0.,0.));
#24298=DIRECTION('ref_axis',(0.,-1.,0.));
#24299=DIRECTION('',(-1.,0.,0.));
#24300=DIRECTION('',(1.,0.,0.));
#24301=DIRECTION('center_axis',(0.,1.,0.));
#24302=DIRECTION('ref_axis',(0.999898028249439,0.,-0.0142805147975766));
#24303=DIRECTION('center_axis',(0.,-1.,0.));
#24304=DIRECTION('ref_axis',(1.,0.,0.));
#24305=DIRECTION('center_axis',(0.,1.,0.));
#24306=DIRECTION('ref_axis',(1.,0.,0.));
#24307=DIRECTION('center_axis',(-0.707106781186548,0.,-0.707106781186548));
#24308=DIRECTION('ref_axis',(0.500000000000005,-0.707106781186541,-0.500000000000005));
#24309=DIRECTION('',(-0.707106781186547,0.,-0.707106781186547));
#24310=DIRECTION('center_axis',(0.855572029308629,0.,0.517683786364528));
#24311=DIRECTION('ref_axis',(-0.517683786364528,0.,0.855572029308629));
#24312=DIRECTION('',(0.707106781186547,0.,0.707106781186547));
#24313=DIRECTION('center_axis',(-0.95447997803503,0.,-0.298274993135947));
#24314=DIRECTION('ref_axis',(0.2109122703048,-0.707106781186545,-0.674919264975359));
#24315=DIRECTION('',(-0.95447997803503,0.,-0.298274993135947));
#24316=DIRECTION('center_axis',(0.988554494713119,0.,0.150864213723769));
#24317=DIRECTION('ref_axis',(-0.150864213723769,0.,0.988554494713118));
#24318=DIRECTION('',(0.95447997803503,0.,0.298274993135947));
#24319=DIRECTION('center_axis',(0.,0.,1.));
#24320=DIRECTION('ref_axis',(-0.707106781186544,-0.707106781186551,0.));
#24321=DIRECTION('',(0.,0.,1.));
#24322=DIRECTION('center_axis',(-0.70710678118655,0.,0.707106781186546));
#24323=DIRECTION('ref_axis',(-0.707106781186546,0.,-0.707106781186549));
#24324=DIRECTION('center_axis',(-1.,0.,0.));
#24325=DIRECTION('ref_axis',(0.,-0.707106781186548,-0.707106781186548));
#24326=DIRECTION('',(-1.,0.,0.));
#24327=DIRECTION('',(1.,0.,0.));
#24328=DIRECTION('center_axis',(0.,0.,1.));
#24329=DIRECTION('ref_axis',(1.,0.,0.));
#24330=DIRECTION('',(0.,1.,0.));
#24331=DIRECTION('',(1.,0.,0.));
#24332=DIRECTION('center_axis',(0.,1.,0.));
#24333=DIRECTION('ref_axis',(0.,0.,1.));
#24334=DIRECTION('',(0.,1.,0.));
#24335=DIRECTION('center_axis',(0.,1.,0.));
#24336=DIRECTION('ref_axis',(1.,0.,0.));
#24337=DIRECTION('center_axis',(0.707106781186548,0.,-0.707106781186548));
#24338=DIRECTION('ref_axis',(-0.707106781186548,0.,-0.707106781186548));
#24339=DIRECTION('',(0.,1.,0.));
#24340=DIRECTION('',(-0.707106781186547,0.,-0.707106781186547));
#24341=DIRECTION('center_axis',(0.298274993135947,0.,-0.95447997803503));
#24342=DIRECTION('ref_axis',(-0.95447997803503,0.,-0.298274993135947));
#24343=DIRECTION('',(0.,1.,0.));
#24344=DIRECTION('',(-0.95447997803503,0.,-0.298274993135947));
#24345=DIRECTION('center_axis',(0.,0.,-1.));
#24346=DIRECTION('ref_axis',(-1.,0.,0.));
#24347=DIRECTION('',(-1.,0.,0.));
#24348=DIRECTION('center_axis',(0.948683298050514,0.,0.316227766016838));
#24349=DIRECTION('ref_axis',(-0.223606797749977,0.707106781186554,0.670820393249931));
#24350=DIRECTION('',(-0.948683298050514,0.,-0.316227766016838));
#24351=DIRECTION('center_axis',(0.987087457637498,0.,0.160182243006963));
#24352=DIRECTION('ref_axis',(0.160182243006963,0.,-0.987087457637497));
#24353=DIRECTION('center_axis',(0.,1.,0.));
#24354=DIRECTION('ref_axis',(-0.999898028249439,0.,-0.0142805147975755));
#24355=DIRECTION('center_axis',(-1.,0.,0.));
#24356=DIRECTION('ref_axis',(0.,0.,1.));
#24357=DIRECTION('center_axis',(0.,-1.,0.));
#24358=DIRECTION('ref_axis',(-1.,0.,0.));
#24359=DIRECTION('center_axis',(1.,0.,0.));
#24360=DIRECTION('ref_axis',(0.,0.70710678118654,0.707106781186555));
#24361=DIRECTION('',(-1.,0.,0.));
#24362=DIRECTION('center_axis',(-0.707106781186548,0.,0.707106781186548));
#24363=DIRECTION('ref_axis',(-0.500000000000001,0.707106781186546,-0.500000000000001));
#24364=DIRECTION('',(0.707106781186547,0.,-0.707106781186547));
#24365=DIRECTION('center_axis',(-0.855572029308621,0.,0.517683786364541));
#24366=DIRECTION('ref_axis',(-0.517683786364541,0.,-0.855572029308621));
#24367=DIRECTION('center_axis',(-0.95447997803503,0.,0.298274993135947));
#24368=DIRECTION('ref_axis',(-0.210912270304798,0.707106781186552,-0.674919264975352));
#24369=DIRECTION('',(0.95447997803503,0.,-0.298274993135947));
#24370=DIRECTION('center_axis',(-0.988554494713122,0.,0.150864213723747));
#24371=DIRECTION('ref_axis',(-0.150864213723747,0.,-0.988554494713122));
#24372=DIRECTION('center_axis',(-1.,0.,0.));
#24373=DIRECTION('ref_axis',(0.,0.707106781186548,-0.707106781186548));
#24374=DIRECTION('',(1.,0.,0.));
#24375=DIRECTION('center_axis',(0.,1.,0.));
#24376=DIRECTION('ref_axis',(1.,0.,0.));
#24377=DIRECTION('center_axis',(0.,1.,0.));
#24378=DIRECTION('ref_axis',(1.,0.,0.));
#24379=DIRECTION('center_axis',(0.,1.,0.));
#24380=DIRECTION('ref_axis',(1.,0.,0.));
#24381=DIRECTION('center_axis',(0.,1.,0.));
#24382=DIRECTION('ref_axis',(1.,0.,0.));
#24383=DIRECTION('center_axis',(0.,-1.,0.));
#24384=DIRECTION('ref_axis',(0.,0.,-1.));
#24385=DIRECTION('center_axis',(0.,1.,0.));
#24386=DIRECTION('ref_axis',(1.,0.,0.));
#24387=DIRECTION('center_axis',(-1.,0.,0.));
#24388=DIRECTION('ref_axis',(0.,0.,1.));
#24389=DIRECTION('center_axis',(0.,-1.,0.));
#24390=DIRECTION('ref_axis',(1.,0.,0.));
#24391=DIRECTION('center_axis',(0.,-1.,0.));
#24392=DIRECTION('ref_axis',(1.,0.,0.));
#24393=DIRECTION('center_axis',(0.,1.,0.));
#24394=DIRECTION('ref_axis',(1.,0.,0.));
#24395=DIRECTION('center_axis',(0.,-1.,0.));
#24396=DIRECTION('ref_axis',(1.,0.,0.));
#24397=DIRECTION('center_axis',(0.,-1.,0.));
#24398=DIRECTION('ref_axis',(1.,0.,0.));
#24399=DIRECTION('',(0.,1.,0.));
#24400=DIRECTION('center_axis',(0.,1.,0.));
#24401=DIRECTION('ref_axis',(1.,0.,0.));
#24402=DIRECTION('center_axis',(1.,0.,0.));
#24403=DIRECTION('ref_axis',(0.,0.70710678118654,0.707106781186555));
#24404=DIRECTION('center_axis',(-1.,0.,0.));
#24405=DIRECTION('ref_axis',(0.,0.,1.));
#24406=DIRECTION('',(-1.,0.,0.));
#24407=DIRECTION('center_axis',(0.987087457637498,0.,-0.160182243006963));
#24408=DIRECTION('ref_axis',(-0.160182243006963,0.,-0.987087457637497));
#24409=DIRECTION('center_axis',(0.948683298050514,0.,-0.316227766016838));
#24410=DIRECTION('ref_axis',(0.223606797749977,0.707106781186554,0.670820393249931));
#24411=DIRECTION('',(-0.948683298050514,0.,0.316227766016838));
#24412=DIRECTION('center_axis',(0.,0.,1.));
#24413=DIRECTION('ref_axis',(-0.707106781186548,0.707106781186548,0.));
#24414=DIRECTION('',(0.,0.,-1.));
#24415=DIRECTION('center_axis',(-0.707106781186548,0.,0.707106781186548));
#24416=DIRECTION('ref_axis',(-0.707106781186548,0.,-0.707106781186548));
#24417=DIRECTION('center_axis',(-1.,0.,0.));
#24418=DIRECTION('ref_axis',(0.,0.707106781186548,-0.707106781186548));
#24419=DIRECTION('',(1.,0.,0.));
#24420=DIRECTION('center_axis',(-0.988554494713124,0.,-0.150864213723736));
#24421=DIRECTION('ref_axis',(0.150864213723736,0.,-0.988554494713124));
#24422=DIRECTION('center_axis',(-0.95447997803503,0.,-0.298274993135947));
#24423=DIRECTION('ref_axis',(0.210912270304798,0.707106781186552,-0.674919264975352));
#24424=DIRECTION('',(0.95447997803503,0.,0.298274993135947));
#24425=DIRECTION('center_axis',(-0.855572029308614,0.,-0.517683786364553));
#24426=DIRECTION('ref_axis',(0.517683786364553,0.,-0.855572029308614));
#24427=DIRECTION('center_axis',(-0.707106781186548,0.,-0.707106781186548));
#24428=DIRECTION('ref_axis',(0.500000000000005,0.707106781186541,-0.500000000000005));
#24429=DIRECTION('',(0.707106781186547,0.,0.707106781186547));
#24430=DIRECTION('center_axis',(0.,1.,0.));
#24431=DIRECTION('ref_axis',(0.999898028249439,0.,-0.0142805147975766));
#24432=DIRECTION('center_axis',(0.,-1.,0.));
#24433=DIRECTION('ref_axis',(1.,0.,0.));
#24434=DIRECTION('center_axis',(0.,1.,0.));
#24435=DIRECTION('ref_axis',(1.,0.,0.));
#24436=DIRECTION('center_axis',(0.,1.,0.));
#24437=DIRECTION('ref_axis',(1.,0.,0.));
#24438=DIRECTION('center_axis',(0.,1.,0.));
#24439=DIRECTION('ref_axis',(1.,0.,0.));
#24440=DIRECTION('center_axis',(0.,1.,0.));
#24441=DIRECTION('ref_axis',(1.,0.,0.));
#24442=DIRECTION('center_axis',(0.,-1.,0.));
#24443=DIRECTION('ref_axis',(0.,0.,-1.));
#24444=DIRECTION('center_axis',(0.,1.,0.));
#24445=DIRECTION('ref_axis',(1.,0.,0.));
#24446=DIRECTION('center_axis',(-1.,0.,0.));
#24447=DIRECTION('ref_axis',(0.,0.,1.));
#24448=DIRECTION('center_axis',(0.,-1.,0.));
#24449=DIRECTION('ref_axis',(1.,0.,0.));
#24450=DIRECTION('center_axis',(0.,-1.,0.));
#24451=DIRECTION('ref_axis',(1.,0.,0.));
#24452=DIRECTION('center_axis',(0.,1.,0.));
#24453=DIRECTION('ref_axis',(1.,0.,0.));
#24454=DIRECTION('center_axis',(0.,-1.,0.));
#24455=DIRECTION('ref_axis',(1.,0.,0.));
#24456=DIRECTION('center_axis',(0.,-1.,0.));
#24457=DIRECTION('ref_axis',(1.,0.,0.));
#24458=DIRECTION('',(0.,1.,0.));
#24459=DIRECTION('center_axis',(0.,1.,0.));
#24460=DIRECTION('ref_axis',(1.,0.,0.));
#24461=DIRECTION('center_axis',(0.,1.,0.));
#24462=DIRECTION('ref_axis',(0.,0.,1.));
#24463=DIRECTION('center_axis',(-1.,0.,0.));
#24464=DIRECTION('ref_axis',(0.,0.,-1.));
#24465=DIRECTION('center_axis',(0.,1.,0.));
#24466=DIRECTION('ref_axis',(1.,0.,0.));
#24467=DIRECTION('center_axis',(0.,1.,0.));
#24468=DIRECTION('ref_axis',(1.,0.,0.));
#24469=DIRECTION('center_axis',(0.,1.,0.));
#24470=DIRECTION('ref_axis',(1.,0.,0.));
#24471=DIRECTION('',(0.,1.,0.));
#24472=DIRECTION('center_axis',(0.,-1.,0.));
#24473=DIRECTION('ref_axis',(1.,0.,0.));
#24474=DIRECTION('center_axis',(0.,-1.,0.));
#24475=DIRECTION('ref_axis',(1.,0.,0.));
#24476=DIRECTION('center_axis',(0.,-1.,0.));
#24477=DIRECTION('ref_axis',(0.,0.,-1.));
#24478=DIRECTION('center_axis',(-1.,0.,0.));
#24479=DIRECTION('ref_axis',(0.,0.,1.));
#24480=DIRECTION('center_axis',(0.,1.,0.));
#24481=DIRECTION('ref_axis',(0.,0.,1.));
#24482=DIRECTION('center_axis',(-1.,0.,0.));
#24483=DIRECTION('ref_axis',(0.,0.,-1.));
#24484=DIRECTION('center_axis',(0.,1.,0.));
#24485=DIRECTION('ref_axis',(1.,0.,0.));
#24486=DIRECTION('center_axis',(0.,1.,0.));
#24487=DIRECTION('ref_axis',(1.,0.,0.));
#24488=DIRECTION('center_axis',(0.,1.,0.));
#24489=DIRECTION('ref_axis',(1.,0.,0.));
#24490=DIRECTION('',(0.,1.,0.));
#24491=DIRECTION('center_axis',(0.,-1.,0.));
#24492=DIRECTION('ref_axis',(1.,0.,0.));
#24493=DIRECTION('center_axis',(0.,-1.,0.));
#24494=DIRECTION('ref_axis',(1.,0.,0.));
#24495=DIRECTION('center_axis',(0.,-1.,0.));
#24496=DIRECTION('ref_axis',(0.,0.,-1.));
#24497=DIRECTION('center_axis',(-1.,0.,0.));
#24498=DIRECTION('ref_axis',(0.,0.,1.));
#24499=DIRECTION('center_axis',(0.,-1.,0.));
#24500=DIRECTION('ref_axis',(0.,0.,-1.));
#24501=DIRECTION('center_axis',(-1.,0.,0.));
#24502=DIRECTION('ref_axis',(0.,0.,1.));
#24503=DIRECTION('center_axis',(0.,-1.,0.));
#24504=DIRECTION('ref_axis',(1.,0.,0.));
#24505=DIRECTION('center_axis',(0.,-1.,0.));
#24506=DIRECTION('ref_axis',(1.,0.,0.));
#24507=DIRECTION('center_axis',(0.,1.,0.));
#24508=DIRECTION('ref_axis',(1.,0.,0.));
#24509=DIRECTION('center_axis',(0.,1.,0.));
#24510=DIRECTION('ref_axis',(1.,0.,0.));
#24511=DIRECTION('center_axis',(0.,1.,0.));
#24512=DIRECTION('ref_axis',(1.,0.,0.));
#24513=DIRECTION('',(0.,1.,0.));
#24514=DIRECTION('center_axis',(0.,1.,0.));
#24515=DIRECTION('ref_axis',(0.,0.,1.));
#24516=DIRECTION('center_axis',(0.,-1.,0.));
#24517=DIRECTION('ref_axis',(1.,0.,0.));
#24518=DIRECTION('center_axis',(-1.,0.,0.));
#24519=DIRECTION('ref_axis',(0.,0.,-1.));
#24520=DIRECTION('center_axis',(0.,1.,0.));
#24521=DIRECTION('ref_axis',(1.,0.,0.));
#24522=DIRECTION('center_axis',(0.,-1.,0.));
#24523=DIRECTION('ref_axis',(1.,0.,0.));
#24524=DIRECTION('center_axis',(0.,-1.,0.));
#24525=DIRECTION('ref_axis',(0.,0.,-1.));
#24526=DIRECTION('center_axis',(-1.,0.,0.));
#24527=DIRECTION('ref_axis',(0.,0.,1.));
#24528=DIRECTION('center_axis',(0.,-1.,0.));
#24529=DIRECTION('ref_axis',(1.,0.,0.));
#24530=DIRECTION('center_axis',(0.,-1.,0.));
#24531=DIRECTION('ref_axis',(1.,0.,0.));
#24532=DIRECTION('center_axis',(0.,1.,0.));
#24533=DIRECTION('ref_axis',(1.,0.,0.));
#24534=DIRECTION('center_axis',(0.,1.,0.));
#24535=DIRECTION('ref_axis',(1.,0.,0.));
#24536=DIRECTION('center_axis',(0.,1.,0.));
#24537=DIRECTION('ref_axis',(1.,0.,0.));
#24538=DIRECTION('',(0.,1.,0.));
#24539=DIRECTION('center_axis',(0.,1.,0.));
#24540=DIRECTION('ref_axis',(0.,0.,1.));
#24541=DIRECTION('center_axis',(0.,-1.,0.));
#24542=DIRECTION('ref_axis',(1.,0.,0.));
#24543=DIRECTION('center_axis',(-1.,0.,0.));
#24544=DIRECTION('ref_axis',(0.,0.,-1.));
#24545=DIRECTION('center_axis',(0.,1.,0.));
#24546=DIRECTION('ref_axis',(1.,0.,0.));
#24547=DIRECTION('',(-1.,0.,0.));
#24548=DIRECTION('center_axis',(0.,-1.,0.));
#24549=DIRECTION('ref_axis',(1.,0.,0.));
#24550=DIRECTION('center_axis',(0.,-1.,0.));
#24551=DIRECTION('ref_axis',(0.,0.,-1.));
#24552=DIRECTION('center_axis',(-1.,0.,0.));
#24553=DIRECTION('ref_axis',(0.,0.,1.));
#24554=DIRECTION('center_axis',(0.,-1.,0.));
#24555=DIRECTION('ref_axis',(1.,0.,0.));
#24556=DIRECTION('center_axis',(0.,-1.,0.));
#24557=DIRECTION('ref_axis',(1.,0.,0.));
#24558=DIRECTION('center_axis',(0.,1.,0.));
#24559=DIRECTION('ref_axis',(1.,0.,0.));
#24560=DIRECTION('center_axis',(0.,1.,0.));
#24561=DIRECTION('ref_axis',(1.,0.,0.));
#24562=DIRECTION('center_axis',(0.,1.,0.));
#24563=DIRECTION('ref_axis',(1.,0.,0.));
#24564=DIRECTION('',(0.,1.,0.));
#24565=DIRECTION('center_axis',(0.,1.,0.));
#24566=DIRECTION('ref_axis',(0.,0.,1.));
#24567=DIRECTION('center_axis',(-1.,0.,0.));
#24568=DIRECTION('ref_axis',(0.,0.,-1.));
#24569=DIRECTION('center_axis',(0.,-1.,0.));
#24570=DIRECTION('ref_axis',(0.,0.,-1.));
#24571=DIRECTION('center_axis',(-1.,0.,0.));
#24572=DIRECTION('ref_axis',(0.,0.,1.));
#24573=DIRECTION('center_axis',(0.,-1.,0.));
#24574=DIRECTION('ref_axis',(1.,0.,0.));
#24575=DIRECTION('center_axis',(0.,-1.,0.));
#24576=DIRECTION('ref_axis',(1.,0.,0.));
#24577=DIRECTION('center_axis',(0.,1.,0.));
#24578=DIRECTION('ref_axis',(1.,0.,0.));
#24579=DIRECTION('center_axis',(0.,1.,0.));
#24580=DIRECTION('ref_axis',(1.,0.,0.));
#24581=DIRECTION('center_axis',(0.,1.,0.));
#24582=DIRECTION('ref_axis',(1.,0.,0.));
#24583=DIRECTION('',(0.,1.,0.));
#24584=DIRECTION('center_axis',(0.,1.,0.));
#24585=DIRECTION('ref_axis',(0.,0.,1.));
#24586=DIRECTION('center_axis',(-1.,0.,0.));
#24587=DIRECTION('ref_axis',(0.,0.,-1.));
#24588=DIRECTION('center_axis',(0.,-1.,0.));
#24589=DIRECTION('ref_axis',(0.,0.,-1.));
#24590=DIRECTION('center_axis',(0.,1.,0.));
#24591=DIRECTION('ref_axis',(1.,0.,0.));
#24592=DIRECTION('center_axis',(-1.,0.,0.));
#24593=DIRECTION('ref_axis',(0.,0.,1.));
#24594=DIRECTION('center_axis',(0.,-1.,0.));
#24595=DIRECTION('ref_axis',(1.,0.,0.));
#24596=DIRECTION('center_axis',(0.,-1.,0.));
#24597=DIRECTION('ref_axis',(1.,0.,0.));
#24598=DIRECTION('center_axis',(0.,1.,0.));
#24599=DIRECTION('ref_axis',(1.,0.,0.));
#24600=DIRECTION('center_axis',(0.,1.,0.));
#24601=DIRECTION('ref_axis',(1.,0.,0.));
#24602=DIRECTION('center_axis',(0.,1.,0.));
#24603=DIRECTION('ref_axis',(1.,0.,0.));
#24604=DIRECTION('',(0.,1.,0.));
#24605=DIRECTION('center_axis',(0.,1.,0.));
#24606=DIRECTION('ref_axis',(0.,0.,1.));
#24607=DIRECTION('',(0.707106781186547,0.,-0.707106781186548));
#24608=DIRECTION('',(1.,0.,0.));
#24609=DIRECTION('',(-1.,0.,0.));
#24610=DIRECTION('',(0.707106781186547,0.,0.707106781186548));
#24611=DIRECTION('',(1.,0.,0.));
#24612=DIRECTION('center_axis',(0.,1.,0.));
#24613=DIRECTION('ref_axis',(1.,0.,0.));
#24614=DIRECTION('',(0.,0.,1.));
#24615=DIRECTION('',(-1.,0.,0.));
#24616=DIRECTION('',(0.,0.,-1.));
#24617=DIRECTION('',(1.,0.,0.));
#24618=DIRECTION('',(0.,0.,1.));
#24619=DIRECTION('',(-1.,0.,0.));
#24620=DIRECTION('',(0.,0.,-1.));
#24621=DIRECTION('',(1.,0.,0.));
#24622=DIRECTION('center_axis',(-0.707106781186547,0.,0.707106781186548));
#24623=DIRECTION('ref_axis',(-0.500000000000001,0.707106781186546,-0.500000000000001));
#24624=DIRECTION('',(-0.707106781186547,0.,0.707106781186548));
#24625=DIRECTION('center_axis',(0.,0.171341174751248,0.985211754819675));
#24626=DIRECTION('ref_axis',(-0.985636596769451,-0.166382691564751,0.0289361202721306));
#24627=DIRECTION('center_axis',(-0.923879532511285,-5.12856164486977E-15,
0.382683432365094));
#24628=DIRECTION('ref_axis',(-0.382683432365094,-1.23814430785112E-14,-0.923879532511285));
#24629=DIRECTION('center_axis',(-1.,0.,0.));
#24630=DIRECTION('ref_axis',(0.,0.707106781186547,-0.707106781186548));
#24631=DIRECTION('center_axis',(-0.923879532511285,-5.12856164486977E-15,
-0.382683432365094));
#24632=DIRECTION('ref_axis',(0.382683432365094,-1.23814430785109E-14,-0.923879532511285));
#24633=DIRECTION('',(-1.,0.,0.));
#24634=DIRECTION('center_axis',(-0.707106781186547,0.,-0.707106781186548));
#24635=DIRECTION('ref_axis',(0.500000000000001,0.707106781186546,-0.500000000000001));
#24636=DIRECTION('',(-0.707106781186547,0.,-0.707106781186548));
#24637=DIRECTION('center_axis',(-0.707106781186548,0.,-0.707106781186547));
#24638=DIRECTION('ref_axis',(-0.707106781186547,0.,0.707106781186548));
#24639=DIRECTION('',(0.,1.,0.));
#24640=DIRECTION('',(0.707106781186547,0.,-0.707106781186548));
#24641=DIRECTION('center_axis',(0.,0.,-1.));
#24642=DIRECTION('ref_axis',(-1.,0.,0.));
#24643=DIRECTION('',(0.,1.,0.));
#24644=DIRECTION('',(1.,0.,0.));
#24645=DIRECTION('center_axis',(0.707106781186548,0.,-0.707106781186547));
#24646=DIRECTION('ref_axis',(-0.707106781186547,0.,-0.707106781186548));
#24647=DIRECTION('',(0.707106781186547,0.,0.707106781186548));
#24648=DIRECTION('center_axis',(1.,0.,0.));
#24649=DIRECTION('ref_axis',(0.,0.707106781186539,0.707106781186556));
#24650=DIRECTION('center_axis',(0.,1.,0.));
#24651=DIRECTION('ref_axis',(0.,0.,1.));
#24652=DIRECTION('center_axis',(0.,-1.,0.));
#24653=DIRECTION('ref_axis',(1.,0.,0.));
#24654=DIRECTION('center_axis',(-1.,0.,0.));
#24655=DIRECTION('ref_axis',(0.,0.,-1.));
#24656=DIRECTION('center_axis',(0.,1.,0.));
#24657=DIRECTION('ref_axis',(1.,0.,0.));
#24658=DIRECTION('',(-0.707106781186547,0.,0.707106781186548));
#24659=DIRECTION('',(-1.,0.,0.));
#24660=DIRECTION('',(-0.707106781186547,0.,-0.707106781186548));
#24661=DIRECTION('',(0.,0.,-1.));
#24662=DIRECTION('',(1.,0.,0.));
#24663=DIRECTION('',(0.,0.,1.));
#24664=DIRECTION('',(1.,0.,0.));
#24665=DIRECTION('',(0.,0.,-1.));
#24666=DIRECTION('',(1.,0.,0.));
#24667=DIRECTION('',(0.,0.,1.));
#24668=DIRECTION('',(1.,0.,0.));
#24669=DIRECTION('',(0.,0.,-1.));
#24670=DIRECTION('',(1.,0.,0.));
#24671=DIRECTION('',(0.,0.,1.));
#24672=DIRECTION('',(1.,0.,0.));
#24673=DIRECTION('',(0.,0.,-1.));
#24674=DIRECTION('',(1.,0.,0.));
#24675=DIRECTION('',(0.,0.,1.));
#24676=DIRECTION('',(1.,0.,0.));
#24677=DIRECTION('',(0.,0.,-1.));
#24678=DIRECTION('center_axis',(0.,-1.,0.));
#24679=DIRECTION('ref_axis',(1.,0.,0.));
#24680=DIRECTION('center_axis',(-1.,0.,0.));
#24681=DIRECTION('ref_axis',(0.,-0.707106781186539,-0.707106781186556));
#24682=DIRECTION('center_axis',(0.923879532511285,9.37720122241289E-15,
-0.382683432365094));
#24683=DIRECTION('ref_axis',(0.382683432365094,-2.26385663682504E-14,0.923879532511285));
#24684=DIRECTION('center_axis',(0.923879532511289,0.,0.382683432365086));
#24685=DIRECTION('ref_axis',(-0.382683432365086,0.,0.923879532511288));
#24686=DIRECTION('center_axis',(-0.707106781186547,0.,0.707106781186548));
#24687=DIRECTION('ref_axis',(-0.500000000000001,-0.707106781186546,-0.500000000000001));
#24688=DIRECTION('center_axis',(0.,0.,-1.));
#24689=DIRECTION('ref_axis',(0.707106781186548,-0.707106781186547,0.));
#24690=DIRECTION('center_axis',(0.382683432365094,0.,0.923879532511285));
#24691=DIRECTION('ref_axis',(-0.923879532511285,0.,0.382683432365094));
#24692=DIRECTION('center_axis',(-0.707106781186547,0.,-0.707106781186548));
#24693=DIRECTION('ref_axis',(0.500000000000001,-0.707106781186546,-0.500000000000001));
#24694=DIRECTION('center_axis',(0.,1.,0.));
#24695=DIRECTION('ref_axis',(0.,0.,1.));
#24696=DIRECTION('center_axis',(-1.,0.,0.));
#24697=DIRECTION('ref_axis',(0.,0.,-1.));
#24698=DIRECTION('center_axis',(0.,1.,0.));
#24699=DIRECTION('ref_axis',(1.,0.,0.));
#24700=DIRECTION('center_axis',(0.,1.,0.));
#24701=DIRECTION('ref_axis',(1.,0.,0.));
#24702=DIRECTION('center_axis',(0.,1.,0.));
#24703=DIRECTION('ref_axis',(1.,0.,0.));
#24704=DIRECTION('',(0.,1.,0.));
#24705=DIRECTION('center_axis',(0.,-1.,0.));
#24706=DIRECTION('ref_axis',(1.,0.,0.));
#24707=DIRECTION('center_axis',(0.,-1.,0.));
#24708=DIRECTION('ref_axis',(1.,0.,0.));
#24709=DIRECTION('center_axis',(0.,-1.,0.));
#24710=DIRECTION('ref_axis',(0.,0.,-1.));
#24711=DIRECTION('center_axis',(-1.,0.,0.));
#24712=DIRECTION('ref_axis',(0.,0.,1.));
#24713=DIRECTION('center_axis',(0.,0.,-1.));
#24714=DIRECTION('ref_axis',(0.707106781186548,0.707106781186547,0.));
#24715=DIRECTION('center_axis',(-0.707106781186548,0.,-0.707106781186548));
#24716=DIRECTION('ref_axis',(-0.707106781186548,0.,0.707106781186548));
#24717=DIRECTION('',(0.,0.,-1.));
#24718=DIRECTION('center_axis',(-0.707106781186548,0.,0.707106781186548));
#24719=DIRECTION('ref_axis',(0.707106781186548,0.,0.707106781186548));
#24720=DIRECTION('center_axis',(-1.,0.,0.));
#24721=DIRECTION('ref_axis',(0.,0.707106781186555,-0.70710678118654));
#24722=DIRECTION('',(-1.,0.,0.));
#24723=DIRECTION('center_axis',(0.707106781186548,0.,-0.707106781186548));
#24724=DIRECTION('ref_axis',(-0.707106781186548,0.,-0.707106781186548));
#24725=DIRECTION('center_axis',(1.,0.,0.));
#24726=DIRECTION('ref_axis',(0.,0.707106781186547,0.707106781186548));
#24727=DIRECTION('',(1.,0.,0.));
#24728=DIRECTION('center_axis',(-0.707106781186548,0.,-0.707106781186548));
#24729=DIRECTION('ref_axis',(-0.707106781186548,0.,0.707106781186548));
#24730=DIRECTION('center_axis',(0.,0.,1.));
#24731=DIRECTION('ref_axis',(-0.707106781186548,0.707106781186547,0.));
#24732=DIRECTION('',(0.,0.,1.));
#24733=DIRECTION('center_axis',(0.,0.,-1.));
#24734=DIRECTION('ref_axis',(-1.,0.,0.));
#24735=DIRECTION('',(0.,1.,0.));
#24736=DIRECTION('',(-1.,0.,0.));
#24737=DIRECTION('',(0.,1.,0.));
#24738=DIRECTION('center_axis',(-1.,0.,0.));
#24739=DIRECTION('ref_axis',(0.,0.,1.));
#24740=DIRECTION('',(0.,1.,0.));
#24741=DIRECTION('',(0.,0.,1.));
#24742=DIRECTION('center_axis',(0.,0.,1.));
#24743=DIRECTION('ref_axis',(0.707106781186548,-0.707106781186547,0.));
#24744=DIRECTION('center_axis',(0.,0.,1.));
#24745=DIRECTION('ref_axis',(0.707106781186548,-0.707106781186547,0.));
#24746=DIRECTION('center_axis',(-0.707106781186548,0.,0.707106781186548));
#24747=DIRECTION('ref_axis',(-0.707106781186548,0.,-0.707106781186548));
#24748=DIRECTION('center_axis',(-1.,0.,0.));
#24749=DIRECTION('ref_axis',(0.,-0.707106781186547,0.707106781186548));
#24750=DIRECTION('center_axis',(-0.707106781186548,0.,-0.707106781186548));
#24751=DIRECTION('ref_axis',(0.707106781186548,0.,-0.707106781186548));
#24752=DIRECTION('center_axis',(0.,0.,-1.));
#24753=DIRECTION('ref_axis',(-0.707106781186548,-0.707106781186547,0.));
#24754=DIRECTION('center_axis',(0.,0.,1.));
#24755=DIRECTION('ref_axis',(-0.707106781186548,-0.707106781186547,0.));
#24756=DIRECTION('',(0.,0.,-1.));
#24757=DIRECTION('center_axis',(1.,0.,0.));
#24758=DIRECTION('ref_axis',(0.,0.,-1.));
#24759=DIRECTION('',(0.,1.,0.));
#24760=DIRECTION('center_axis',(0.,0.,-1.));
#24761=DIRECTION('ref_axis',(0.707106781186548,0.707106781186547,0.));
#24762=DIRECTION('center_axis',(-0.707106781186548,0.,-0.707106781186548));
#24763=DIRECTION('ref_axis',(-0.707106781186548,0.,0.707106781186548));
#24764=DIRECTION('',(0.,0.,-1.));
#24765=DIRECTION('center_axis',(-0.707106781186548,0.,0.707106781186548));
#24766=DIRECTION('ref_axis',(0.707106781186548,0.,0.707106781186548));
#24767=DIRECTION('center_axis',(-1.,0.,0.));
#24768=DIRECTION('ref_axis',(0.,0.707106781186555,-0.70710678118654));
#24769=DIRECTION('',(-1.,0.,0.));
#24770=DIRECTION('center_axis',(0.707106781186548,0.,-0.707106781186548));
#24771=DIRECTION('ref_axis',(-0.707106781186548,0.,-0.707106781186548));
#24772=DIRECTION('center_axis',(1.,0.,0.));
#24773=DIRECTION('ref_axis',(0.,0.707106781186547,0.707106781186548));
#24774=DIRECTION('',(1.,0.,0.));
#24775=DIRECTION('center_axis',(-0.707106781186548,0.,-0.707106781186548));
#24776=DIRECTION('ref_axis',(-0.707106781186548,0.,0.707106781186548));
#24777=DIRECTION('center_axis',(0.,0.,1.));
#24778=DIRECTION('ref_axis',(-0.707106781186548,0.707106781186547,0.));
#24779=DIRECTION('',(0.,0.,1.));
#24780=DIRECTION('center_axis',(0.,0.,-1.));
#24781=DIRECTION('ref_axis',(-1.,0.,0.));
#24782=DIRECTION('',(0.,1.,0.));
#24783=DIRECTION('',(-1.,0.,0.));
#24784=DIRECTION('',(0.,1.,0.));
#24785=DIRECTION('center_axis',(-1.,0.,0.));
#24786=DIRECTION('ref_axis',(0.,0.,1.));
#24787=DIRECTION('',(0.,1.,0.));
#24788=DIRECTION('',(0.,0.,1.));
#24789=DIRECTION('center_axis',(0.,0.,1.));
#24790=DIRECTION('ref_axis',(0.707106781186548,-0.707106781186547,0.));
#24791=DIRECTION('center_axis',(0.,0.,1.));
#24792=DIRECTION('ref_axis',(0.707106781186548,-0.707106781186547,0.));
#24793=DIRECTION('center_axis',(-0.707106781186548,0.,0.707106781186548));
#24794=DIRECTION('ref_axis',(-0.707106781186548,0.,-0.707106781186548));
#24795=DIRECTION('center_axis',(-1.,0.,0.));
#24796=DIRECTION('ref_axis',(0.,-0.707106781186547,0.707106781186548));
#24797=DIRECTION('center_axis',(-0.707106781186548,0.,-0.707106781186548));
#24798=DIRECTION('ref_axis',(0.707106781186548,0.,-0.707106781186548));
#24799=DIRECTION('center_axis',(0.,0.,-1.));
#24800=DIRECTION('ref_axis',(-0.707106781186548,-0.707106781186547,0.));
#24801=DIRECTION('center_axis',(0.,0.,1.));
#24802=DIRECTION('ref_axis',(-0.707106781186548,-0.707106781186547,0.));
#24803=DIRECTION('',(0.,0.,-1.));
#24804=DIRECTION('center_axis',(1.,0.,0.));
#24805=DIRECTION('ref_axis',(0.,0.,-1.));
#24806=DIRECTION('',(0.,1.,0.));
#24807=DIRECTION('center_axis',(0.,0.,-1.));
#24808=DIRECTION('ref_axis',(-0.707106781186548,-0.707106781186547,0.));
#24809=DIRECTION('center_axis',(0.,0.,1.));
#24810=DIRECTION('ref_axis',(-0.707106781186548,-0.707106781186547,0.));
#24811=DIRECTION('',(0.,0.,1.));
#24812=DIRECTION('center_axis',(0.,0.,-1.));
#24813=DIRECTION('ref_axis',(-0.707106781186548,-0.707106781186547,0.));
#24814=DIRECTION('',(0.,0.,-1.));
#24815=DIRECTION('center_axis',(0.,0.,1.));
#24816=DIRECTION('ref_axis',(-0.707106781186548,-0.707106781186547,0.));
#24817=DIRECTION('',(0.,0.,-1.));
#24818=DIRECTION('center_axis',(0.,0.,-1.));
#24819=DIRECTION('ref_axis',(-0.707106781186548,0.707106781186547,0.));
#24820=DIRECTION('center_axis',(0.,0.,1.));
#24821=DIRECTION('ref_axis',(-0.707106781186548,0.707106781186547,0.));
#24822=DIRECTION('',(0.,0.,-1.));
#24823=DIRECTION('center_axis',(0.,0.,1.));
#24824=DIRECTION('ref_axis',(-0.707106781186548,0.707106781186547,0.));
#24825=DIRECTION('center_axis',(0.,0.,1.));
#24826=DIRECTION('ref_axis',(1.,0.,0.));
#24827=DIRECTION('',(0.,-1.,0.));
#24828=DIRECTION('center_axis',(0.,0.,1.));
#24829=DIRECTION('ref_axis',(0.707106781186548,-0.707106781186547,0.));
#24830=DIRECTION('center_axis',(0.,0.,1.));
#24831=DIRECTION('ref_axis',(0.707106781186548,0.707106781186547,0.));
#24832=DIRECTION('',(1.,0.,0.));
#24833=DIRECTION('',(0.,1.,0.));
#24834=DIRECTION('center_axis',(-1.,0.,0.));
#24835=DIRECTION('ref_axis',(0.,0.,-1.));
#24836=DIRECTION('',(0.,-1.,0.));
#24837=DIRECTION('center_axis',(0.,0.,-1.));
#24838=DIRECTION('ref_axis',(1.,0.,0.));
#24839=DIRECTION('',(1.,0.,0.));
#24840=DIRECTION('center_axis',(0.,0.,1.));
#24841=DIRECTION('ref_axis',(0.707106781186548,0.707106781186547,0.));
#24842=DIRECTION('center_axis',(0.,0.,1.));
#24843=DIRECTION('ref_axis',(0.707106781186548,-0.707106781186547,0.));
#24844=DIRECTION('',(1.,0.,0.));
#24845=DIRECTION('center_axis',(0.,0.,1.));
#24846=DIRECTION('ref_axis',(0.707106781186548,-0.707106781186547,0.));
#24847=DIRECTION('center_axis',(0.,0.,-1.));
#24848=DIRECTION('ref_axis',(0.707106781186548,-0.707106781186547,0.));
#24849=DIRECTION('',(0.,0.,-1.));
#24850=DIRECTION('',(0.,0.,1.));
#24851=DIRECTION('',(0.,0.,1.));
#24852=DIRECTION('center_axis',(0.,-1.,0.));
#24853=DIRECTION('ref_axis',(0.,0.,-1.));
#24854=DIRECTION('',(-1.,0.,0.));
#24855=DIRECTION('center_axis',(0.,0.,1.));
#24856=DIRECTION('ref_axis',(-1.,0.,0.));
#24857=DIRECTION('',(0.,-1.,0.));
#24858=DIRECTION('center_axis',(1.,0.,0.));
#24859=DIRECTION('ref_axis',(0.,0.,1.));
#24860=DIRECTION('center_axis',(0.,0.,1.));
#24861=DIRECTION('ref_axis',(0.707106781186548,0.707106781186547,0.));
#24862=DIRECTION('',(0.,0.,1.));
#24863=DIRECTION('center_axis',(0.,0.,-1.));
#24864=DIRECTION('ref_axis',(-0.707106781186548,-0.707106781186547,0.));
#24865=DIRECTION('center_axis',(0.,0.,1.));
#24866=DIRECTION('ref_axis',(-0.707106781186548,-0.707106781186547,0.));
#24867=DIRECTION('',(0.,0.,1.));
#24868=DIRECTION('center_axis',(0.,0.,-1.));
#24869=DIRECTION('ref_axis',(-0.707106781186548,-0.707106781186547,0.));
#24870=DIRECTION('',(0.,0.,-1.));
#24871=DIRECTION('center_axis',(0.,0.,1.));
#24872=DIRECTION('ref_axis',(-0.707106781186548,-0.707106781186547,0.));
#24873=DIRECTION('',(0.,0.,-1.));
#24874=DIRECTION('center_axis',(0.,0.,-1.));
#24875=DIRECTION('ref_axis',(-0.707106781186548,0.707106781186547,0.));
#24876=DIRECTION('center_axis',(0.,0.,1.));
#24877=DIRECTION('ref_axis',(-0.707106781186548,0.707106781186547,0.));
#24878=DIRECTION('',(0.,0.,-1.));
#24879=DIRECTION('center_axis',(0.,0.,1.));
#24880=DIRECTION('ref_axis',(-0.707106781186548,0.707106781186547,0.));
#24881=DIRECTION('center_axis',(0.,0.,1.));
#24882=DIRECTION('ref_axis',(1.,0.,0.));
#24883=DIRECTION('',(0.,-1.,0.));
#24884=DIRECTION('center_axis',(0.,0.,1.));
#24885=DIRECTION('ref_axis',(0.707106781186548,-0.707106781186547,0.));
#24886=DIRECTION('center_axis',(0.,0.,1.));
#24887=DIRECTION('ref_axis',(0.707106781186548,0.707106781186547,0.));
#24888=DIRECTION('',(1.,0.,0.));
#24889=DIRECTION('',(0.,1.,0.));
#24890=DIRECTION('center_axis',(-1.,0.,0.));
#24891=DIRECTION('ref_axis',(0.,0.,-1.));
#24892=DIRECTION('',(0.,-1.,0.));
#24893=DIRECTION('center_axis',(0.,0.,-1.));
#24894=DIRECTION('ref_axis',(1.,0.,0.));
#24895=DIRECTION('',(1.,0.,0.));
#24896=DIRECTION('center_axis',(0.,0.,1.));
#24897=DIRECTION('ref_axis',(0.707106781186548,0.707106781186547,0.));
#24898=DIRECTION('center_axis',(0.,0.,1.));
#24899=DIRECTION('ref_axis',(0.707106781186548,-0.707106781186547,0.));
#24900=DIRECTION('',(1.,0.,0.));
#24901=DIRECTION('center_axis',(0.,0.,1.));
#24902=DIRECTION('ref_axis',(0.707106781186548,-0.707106781186547,0.));
#24903=DIRECTION('center_axis',(0.,0.,-1.));
#24904=DIRECTION('ref_axis',(0.707106781186548,-0.707106781186547,0.));
#24905=DIRECTION('',(0.,0.,-1.));
#24906=DIRECTION('',(0.,0.,1.));
#24907=DIRECTION('',(0.,0.,1.));
#24908=DIRECTION('center_axis',(0.,-1.,0.));
#24909=DIRECTION('ref_axis',(0.,0.,-1.));
#24910=DIRECTION('',(-1.,0.,0.));
#24911=DIRECTION('center_axis',(0.,0.,1.));
#24912=DIRECTION('ref_axis',(-1.,0.,0.));
#24913=DIRECTION('',(0.,-1.,0.));
#24914=DIRECTION('center_axis',(1.,0.,0.));
#24915=DIRECTION('ref_axis',(0.,0.,1.));
#24916=DIRECTION('center_axis',(0.,0.,1.));
#24917=DIRECTION('ref_axis',(0.707106781186548,0.707106781186547,0.));
#24918=DIRECTION('',(0.,0.,1.));
#24919=DIRECTION('center_axis',(0.,1.,0.));
#24920=DIRECTION('ref_axis',(1.,0.,0.));
#24921=DIRECTION('center_axis',(0.,1.,0.));
#24922=DIRECTION('ref_axis',(1.,0.,0.));
#24923=DIRECTION('center_axis',(0.,0.,1.));
#24924=DIRECTION('ref_axis',(0.,1.,0.));
#24925=DIRECTION('center_axis',(0.,-0.171341174751248,-0.985211754819675));
#24926=DIRECTION('ref_axis',(0.,-0.985211754819675,0.171341174751248));
#24927=DIRECTION('center_axis',(0.,0.,-1.));
#24928=DIRECTION('ref_axis',(0.,1.,0.));
#60100=CARTESIAN_POINT('',(0.,0.,0.));
#60101=CARTESIAN_POINT('Origin',(-18.368,7.548,38.36));
#60102=CARTESIAN_POINT('',(-18.768,14.272,38.36));
#60103=CARTESIAN_POINT('',(-18.768,8.576,38.36));
#60104=CARTESIAN_POINT('',(-18.768,7.548,38.36));
#60105=CARTESIAN_POINT('',(-18.368,8.976,38.76));
#60106=CARTESIAN_POINT('Origin',(-18.368,8.576,38.36));
#60107=CARTESIAN_POINT('',(-18.368,13.872,38.76));
#60108=CARTESIAN_POINT('',(-18.368,7.548,38.76));
#60109=CARTESIAN_POINT('Origin',(-18.368,14.272,38.36));
#60110=CARTESIAN_POINT('Origin',(-18.368,8.576,37.332));
#60111=CARTESIAN_POINT('',(-18.368,8.976,41.616));
#60112=CARTESIAN_POINT('',(-18.368,8.976,37.332));
#60113=CARTESIAN_POINT('',(-18.768,8.576,42.016));
#60114=CARTESIAN_POINT('',(-18.768,8.576,37.332));
#60115=CARTESIAN_POINT('Origin',(-18.368,8.576,42.016));
#60116=CARTESIAN_POINT('Origin',(-18.368,14.272,38.76));
#60117=CARTESIAN_POINT('',(-18.768,14.272,42.016));
#60118=CARTESIAN_POINT('',(-18.768,14.272,38.76));
#60119=CARTESIAN_POINT('',(-18.368,13.872,41.616));
#60120=CARTESIAN_POINT('',(-18.368,13.872,38.76));
#60121=CARTESIAN_POINT('Origin',(-18.368,14.272,42.016));
#60122=CARTESIAN_POINT('Origin',(-18.368,5.1,42.016));
#60123=CARTESIAN_POINT('',(-18.768,5.1,42.016));
#60124=CARTESIAN_POINT('',(-18.368,5.1,41.616));
#60125=CARTESIAN_POINT('Origin',(-17.544,13.872,41.616));
#60126=CARTESIAN_POINT('',(-17.944,13.872,38.76));
#60127=CARTESIAN_POINT('',(-17.544,13.872,38.76));
#60128=CARTESIAN_POINT('',(-17.944,13.872,41.616));
#60129=CARTESIAN_POINT('',(-17.944,13.872,40.392));
#60130=CARTESIAN_POINT('',(-17.544,13.872,41.616));
#60131=CARTESIAN_POINT('Origin',(-17.544,13.872,38.76));
#60132=CARTESIAN_POINT('',(-17.944,8.976,38.76));
#60133=CARTESIAN_POINT('',(-17.544,8.976,38.76));
#60134=CARTESIAN_POINT('',(-17.944,12.852,38.76));
#60135=CARTESIAN_POINT('Origin',(-18.768,1.224,35.904));
#60136=CARTESIAN_POINT('',(-18.768,2.4322958752602,36.3127352401262));
#60137=CARTESIAN_POINT('',(-18.768,21.216,33.0460040879975));
#60138=CARTESIAN_POINT('',(-18.768,11.3065034423776,34.769394793671));
#60139=CARTESIAN_POINT('',(-18.768,2.048,35.904));
#60140=CARTESIAN_POINT('Origin',(-18.768,2.048,36.4696854249492));
#60141=CARTESIAN_POINT('',(-18.768,1.624,35.904));
#60142=CARTESIAN_POINT('',(-18.768,1.224,35.904));
#60143=CARTESIAN_POINT('',(-18.768,1.624,45.296));
#60144=CARTESIAN_POINT('',(-18.768,1.624,37.74));
#60145=CARTESIAN_POINT('',(-18.768,21.216,45.296));
#60146=CARTESIAN_POINT('',(-18.768,1.224,45.296));
#60147=CARTESIAN_POINT('',(-18.768,21.216,32.64));
#60148=CARTESIAN_POINT('Origin',(-18.368,11.3065034423776,34.769394793671));
#60149=CARTESIAN_POINT('',(-18.368,2.43108893861255,35.9069410541543));
#60150=CARTESIAN_POINT('Ctrl Pts',(-18.768,2.43229587526021,36.3127352401262));
#60151=CARTESIAN_POINT('Ctrl Pts',(-18.768,2.43163865325589,36.3095167959342));
#60152=CARTESIAN_POINT('Ctrl Pts',(-18.7679595430623,2.43096733281414,36.3062986618292));
#60153=CARTESIAN_POINT('Ctrl Pts',(-18.7670365475227,2.42318946934172,36.2696281280777));
#60154=CARTESIAN_POINT('Ctrl Pts',(-18.7617623197712,2.41476971759224,36.2363087583245));
#60155=CARTESIAN_POINT('Ctrl Pts',(-18.7426520469775,2.39907273991872,36.1720724010591));
#60156=CARTESIAN_POINT('Ctrl Pts',(-18.7287849670363,2.3918106985706,36.1410603177669));
#60157=CARTESIAN_POINT('Ctrl Pts',(-18.6936954523635,2.38175700469627,36.0832890660283));
#60158=CARTESIAN_POINT('Ctrl Pts',(-18.672468995915,2.37899329807783,36.0565274804843));
#60159=CARTESIAN_POINT('Ctrl Pts',(-18.6001051985816,2.37899329807783,35.9841636831509));
#60160=CARTESIAN_POINT('Ctrl Pts',(-18.5389719289432,2.39142035091093,35.9463799403922));
#60161=CARTESIAN_POINT('Ctrl Pts',(-18.4407068959515,2.41470336343454,35.9150691173314));
#60162=CARTESIAN_POINT('Ctrl Pts',(-18.4068151443652,2.42301155359813,35.9087870732679));
#60163=CARTESIAN_POINT('Ctrl Pts',(-18.3711843766952,2.43043368046293,35.9070646745485));
#60164=CARTESIAN_POINT('Ctrl Pts',(-18.3695923051444,2.43076276515015,35.9069977799739));
#60165=CARTESIAN_POINT('Ctrl Pts',(-18.368,2.43108893861256,35.9069410541544));
#60166=CARTESIAN_POINT('',(-18.368,21.216,32.64));
#60167=CARTESIAN_POINT('Origin',(-18.368,21.216,33.0460040879975));
#60168=CARTESIAN_POINT('',(-18.368,11.2379669724771,34.3753100917431));
#60169=CARTESIAN_POINT('Origin',(-17.944,10.404,42.016));
#60170=CARTESIAN_POINT('',(-17.544,14.272,42.016));
#60171=CARTESIAN_POINT('',(-17.544,8.576,42.016));
#60172=CARTESIAN_POINT('',(-17.544,10.404,42.016));
#60173=CARTESIAN_POINT('',(-17.944,8.976,41.616));
#60174=CARTESIAN_POINT('Origin',(-17.944,8.576,42.016));
#60175=CARTESIAN_POINT('',(-17.944,10.404,41.616));
#60176=CARTESIAN_POINT('Origin',(-17.944,14.272,42.016));
#60177=CARTESIAN_POINT('Origin',(-17.944,12.852,38.36));
#60178=CARTESIAN_POINT('',(-17.544,8.576,38.36));
#60179=CARTESIAN_POINT('',(-17.544,14.272,38.36));
#60180=CARTESIAN_POINT('',(-17.544,12.852,38.36));
#60181=CARTESIAN_POINT('Origin',(-17.944,14.272,38.36));
#60182=CARTESIAN_POINT('Origin',(-17.944,8.576,38.36));
#60183=CARTESIAN_POINT('Origin',(-17.944,14.272,40.392));
#60184=CARTESIAN_POINT('',(-17.544,14.272,40.392));
#60185=CARTESIAN_POINT('Origin',(-17.944,8.576,38.964));
#60186=CARTESIAN_POINT('',(-17.544,8.576,38.964));
#60187=CARTESIAN_POINT('',(-17.944,8.976,38.964));
#60188=CARTESIAN_POINT('Origin',(-17.544,8.976,38.76));
#60189=CARTESIAN_POINT('',(-17.544,8.976,41.616));
#60190=CARTESIAN_POINT('Origin',(-17.544,11.832,39.168));
#60191=CARTESIAN_POINT('',(-17.544,21.616,32.9764388706062));
#60192=CARTESIAN_POINT('',(-17.544,2.448,36.3100040879975));
#60193=CARTESIAN_POINT('',(-17.544,16.179296102928,33.9219525918361));
#60194=CARTESIAN_POINT('',(-17.544,21.616,21.216));
#60195=CARTESIAN_POINT('',(-17.544,21.616,36.312));
#60196=CARTESIAN_POINT('',(-17.544,22.04,21.216));
#60197=CARTESIAN_POINT('',(-17.544,21.216,21.216));
#60198=CARTESIAN_POINT('',(-17.544,22.04,45.296));
#60199=CARTESIAN_POINT('',(-17.544,22.04,36.312));
#60200=CARTESIAN_POINT('',(-17.544,2.448,45.296));
#60201=CARTESIAN_POINT('',(-17.544,6.528,45.296));
#60202=CARTESIAN_POINT('',(-17.544,2.448,39.372));
#60203=CARTESIAN_POINT('Origin',(-17.944,16.179296102928,33.9219525918361));
#60204=CARTESIAN_POINT('',(-17.944,21.216,32.64));
#60205=CARTESIAN_POINT('Origin',(-17.944,21.616,32.9764388706062));
#60206=CARTESIAN_POINT('',(-17.944,2.448,35.904));
#60207=CARTESIAN_POINT('Origin',(-17.944,2.448,36.3100040879975));
#60208=CARTESIAN_POINT('',(-17.944,16.1107596330275,33.5278678899083));
#60209=CARTESIAN_POINT('Origin',(18.368,1.09602270843261,36.5451305734875));
#60210=CARTESIAN_POINT('',(18.768,2.4322958752602,36.3127352401262));
#60211=CARTESIAN_POINT('',(18.368,2.43108893861254,35.9069410541543));
#60212=CARTESIAN_POINT('Ctrl Pts',(18.368,2.43108893861255,35.9069410541543));
#60213=CARTESIAN_POINT('Ctrl Pts',(18.3695923051444,2.43076276515014,35.9069977799739));
#60214=CARTESIAN_POINT('Ctrl Pts',(18.3711843766952,2.43043368046293,35.9070646745484));
#60215=CARTESIAN_POINT('Ctrl Pts',(18.4068151443652,2.42301155359813,35.9087870732679));
#60216=CARTESIAN_POINT('Ctrl Pts',(18.4407068959515,2.41470336343453,35.9150691173314));
#60217=CARTESIAN_POINT('Ctrl Pts',(18.5389719289432,2.39142035091092,35.9463799403922));
#60218=CARTESIAN_POINT('Ctrl Pts',(18.6001051985816,2.37899329807782,35.9841636831509));
#60219=CARTESIAN_POINT('Ctrl Pts',(18.672468995915,2.37899329807782,36.0565274804843));
#60220=CARTESIAN_POINT('Ctrl Pts',(18.6936954523635,2.38175700469626,36.0832890660283));
#60221=CARTESIAN_POINT('Ctrl Pts',(18.7287849670363,2.3918106985706,36.1410603177669));
#60222=CARTESIAN_POINT('Ctrl Pts',(18.7426520469775,2.39907273991871,36.1720724010591));
#60223=CARTESIAN_POINT('Ctrl Pts',(18.7617623197712,2.41476971759224,36.2363087583245));
#60224=CARTESIAN_POINT('Ctrl Pts',(18.7670365475227,2.42318946934172,36.2696281280776));
#60225=CARTESIAN_POINT('Ctrl Pts',(18.7679595430623,2.43096733281413,36.3062986618292));
#60226=CARTESIAN_POINT('Ctrl Pts',(18.768,2.4316386532559,36.3095167959342));
#60227=CARTESIAN_POINT('Ctrl Pts',(18.768,2.43229587526021,36.3127352401262));
#60228=CARTESIAN_POINT('',(18.368,21.216,32.64));
#60229=CARTESIAN_POINT('',(18.368,1.02748623853211,36.1510458715596));
#60230=CARTESIAN_POINT('',(18.768,21.216,33.0460040879975));
#60231=CARTESIAN_POINT('Origin',(18.368,21.216,33.0460040879975));
#60232=CARTESIAN_POINT('',(18.768,1.09602270843261,36.5451305734875));
#60233=CARTESIAN_POINT('Origin',(17.544,2.448,35.904));
#60234=CARTESIAN_POINT('',(18.2023145750508,2.448,35.904));
#60235=CARTESIAN_POINT('Origin',(18.2718797924421,2.048,35.9735652173913));
#60236=CARTESIAN_POINT('',(17.944,2.448,35.904));
#60237=CARTESIAN_POINT('',(8.772,2.448,35.904));
#60238=CARTESIAN_POINT('',(17.944,21.216,32.64));
#60239=CARTESIAN_POINT('',(17.944,6.72675963302752,35.1598678899083));
#60240=CARTESIAN_POINT('',(17.544,21.216,32.64));
#60241=CARTESIAN_POINT('Origin',(18.368,7.548,42.016));
#60242=CARTESIAN_POINT('',(18.768,14.272,42.016));
#60243=CARTESIAN_POINT('',(18.768,8.576,42.016));
#60244=CARTESIAN_POINT('',(18.768,7.548,42.016));
#60245=CARTESIAN_POINT('',(18.368,8.976,41.616));
#60246=CARTESIAN_POINT('Origin',(18.368,8.576,42.016));
#60247=CARTESIAN_POINT('',(18.368,13.872,41.616));
#60248=CARTESIAN_POINT('',(18.368,7.548,41.616));
#60249=CARTESIAN_POINT('Origin',(18.368,14.272,42.016));
#60250=CARTESIAN_POINT('Origin',(18.368,8.576,43.656));
#60251=CARTESIAN_POINT('',(18.368,8.976,38.76));
#60252=CARTESIAN_POINT('',(18.368,8.976,43.656));
#60253=CARTESIAN_POINT('',(18.768,8.576,38.36));
#60254=CARTESIAN_POINT('',(18.768,8.576,43.656));
#60255=CARTESIAN_POINT('Origin',(18.368,8.576,38.36));
#60256=CARTESIAN_POINT('Origin',(18.368,14.272,42.228));
#60257=CARTESIAN_POINT('',(18.768,14.272,38.36));
#60258=CARTESIAN_POINT('',(18.768,14.272,42.228));
#60259=CARTESIAN_POINT('',(18.368,13.872,38.76));
#60260=CARTESIAN_POINT('',(18.368,13.872,42.228));
#60261=CARTESIAN_POINT('Origin',(18.368,14.272,38.36));
#60262=CARTESIAN_POINT('Origin',(18.368,5.1,38.36));
#60263=CARTESIAN_POINT('',(18.768,5.1,38.36));
#60264=CARTESIAN_POINT('',(18.368,5.1,38.76));
#60265=CARTESIAN_POINT('Origin',(17.544,13.872,38.76));
#60266=CARTESIAN_POINT('',(17.944,13.872,41.616));
#60267=CARTESIAN_POINT('',(17.544,13.872,41.616));
#60268=CARTESIAN_POINT('',(17.944,13.872,38.76));
#60269=CARTESIAN_POINT('',(17.944,13.872,38.964));
#60270=CARTESIAN_POINT('',(17.544,13.872,38.76));
#60271=CARTESIAN_POINT('Origin',(17.544,13.872,41.616));
#60272=CARTESIAN_POINT('',(17.944,8.976,41.616));
#60273=CARTESIAN_POINT('',(17.544,8.976,41.616));
#60274=CARTESIAN_POINT('',(17.944,12.852,41.616));
#60275=CARTESIAN_POINT('Origin',(18.768,1.224,45.696));
#60276=CARTESIAN_POINT('',(18.768,21.216,45.296));
#60277=CARTESIAN_POINT('',(18.768,21.216,32.64));
#60278=CARTESIAN_POINT('',(18.768,1.624,45.296));
#60279=CARTESIAN_POINT('',(18.768,1.224,45.296));
#60280=CARTESIAN_POINT('',(18.768,1.624,35.904));
#60281=CARTESIAN_POINT('',(18.768,1.624,42.636));
#60282=CARTESIAN_POINT('',(18.768,2.048,35.904));
#60283=CARTESIAN_POINT('',(18.768,1.224,35.904));
#60284=CARTESIAN_POINT('Origin',(18.768,2.048,36.4696854249492));
#60285=CARTESIAN_POINT('Origin',(-17.944,22.04,45.296));
#60286=CARTESIAN_POINT('',(-17.944,22.04,45.696));
#60287=CARTESIAN_POINT('Origin',(-17.944,22.04,45.296));
#60288=CARTESIAN_POINT('',(-17.944,22.44,45.296));
#60289=CARTESIAN_POINT('Origin',(-17.944,22.04,45.296));
#60290=CARTESIAN_POINT('Origin',(-17.944,22.04,45.296));
#60291=CARTESIAN_POINT('Origin',(-17.944,6.528,45.296));
#60292=CARTESIAN_POINT('',(-17.944,2.048,45.696));
#60293=CARTESIAN_POINT('Origin',(-17.944,2.048,45.296));
#60294=CARTESIAN_POINT('',(-17.944,6.528,45.696));
#60295=CARTESIAN_POINT('Origin',(-18.768,1.224,45.696));
#60296=CARTESIAN_POINT('',(17.944,2.048,45.696));
#60297=CARTESIAN_POINT('',(-9.384,2.048,45.696));
#60298=CARTESIAN_POINT('',(-32.64,22.04,45.696));
#60299=CARTESIAN_POINT('',(-26.316,22.04,45.696));
#60300=CARTESIAN_POINT('',(-32.64,21.616,45.696));
#60301=CARTESIAN_POINT('',(-32.64,21.216,45.696));
#60302=CARTESIAN_POINT('',(-18.368,21.616,45.696));
#60303=CARTESIAN_POINT('',(-26.316,21.616,45.696));
#60304=CARTESIAN_POINT('',(-18.368,1.624,45.696));
#60305=CARTESIAN_POINT('',(-18.368,1.224,45.696));
#60306=CARTESIAN_POINT('',(18.368,1.624,45.696));
#60307=CARTESIAN_POINT('',(-9.384,1.624,45.696));
#60308=CARTESIAN_POINT('',(18.368,21.616,45.696));
#60309=CARTESIAN_POINT('',(18.368,1.224,45.696));
#60310=CARTESIAN_POINT('',(32.64,21.616,45.696));
#60311=CARTESIAN_POINT('',(7.548,21.616,45.696));
#60312=CARTESIAN_POINT('',(32.64,22.04,45.696));
#60313=CARTESIAN_POINT('',(32.64,21.216,45.696));
#60314=CARTESIAN_POINT('',(17.944,22.04,45.696));
#60315=CARTESIAN_POINT('',(7.548,22.04,45.696));
#60316=CARTESIAN_POINT('',(17.944,6.528,45.696));
#60317=CARTESIAN_POINT('Origin',(-26.316,22.04,45.296));
#60318=CARTESIAN_POINT('',(-32.5750889359327,22.44,45.296));
#60319=CARTESIAN_POINT('',(-26.316,22.44,45.296));
#60320=CARTESIAN_POINT('Origin',(-32.5750889359327,22.04,45.296));
#60321=CARTESIAN_POINT('Origin',(-17.944,22.04,36.312));
#60322=CARTESIAN_POINT('',(-17.944,22.44,21.616));
#60323=CARTESIAN_POINT('Origin',(-17.944,22.04,21.616));
#60324=CARTESIAN_POINT('',(-17.944,22.44,36.312));
#60325=CARTESIAN_POINT('Origin',(7.548,21.616,45.296));
#60326=CARTESIAN_POINT('Origin',(18.368,21.616,45.296));
#60327=CARTESIAN_POINT('',(32.5750889359327,21.216,45.296));
#60328=CARTESIAN_POINT('',(7.548,21.216,45.296));
#60329=CARTESIAN_POINT('Origin',(32.5750889359326,21.616,45.296));
#60330=CARTESIAN_POINT('Origin',(18.368,1.624,45.296));
#60331=CARTESIAN_POINT('Origin',(18.368,1.624,45.296));
#60332=CARTESIAN_POINT('',(18.368,1.224,45.296));
#60333=CARTESIAN_POINT('Origin',(18.368,1.624,45.296));
#60334=CARTESIAN_POINT('Origin',(18.368,1.624,45.296));
#60335=CARTESIAN_POINT('Origin',(18.368,1.224,45.296));
#60336=CARTESIAN_POINT('Origin',(34.9003088935933,21.616,44.5209266807798));
#60337=CARTESIAN_POINT('',(37.4710889359326,21.216,43.664));
#60338=CARTESIAN_POINT('',(34.9003088935933,21.216,44.5209266807798));
#60339=CARTESIAN_POINT('',(37.536,21.616,44.064));
#60340=CARTESIAN_POINT('Origin',(37.4710889359326,21.616,43.664));
#60341=CARTESIAN_POINT('',(35.0268,21.616,44.9004));
#60342=CARTESIAN_POINT('Origin',(32.64,21.216,45.696));
#60343=CARTESIAN_POINT('',(37.536,22.04,44.064));
#60344=CARTESIAN_POINT('',(37.536,21.216,44.064));
#60345=CARTESIAN_POINT('',(35.0268,22.04,44.9004));
#60346=CARTESIAN_POINT('Origin',(-17.944,21.616,36.312));
#60347=CARTESIAN_POINT('',(-17.944,21.216,21.616));
#60348=CARTESIAN_POINT('',(-17.944,21.216,36.312));
#60349=CARTESIAN_POINT('Origin',(-17.944,21.616,21.616));
#60350=CARTESIAN_POINT('Origin',(-25.704,21.616,21.616));
#60351=CARTESIAN_POINT('',(-24.4189556308608,21.216,21.616));
#60352=CARTESIAN_POINT('',(-25.704,21.216,21.616));
#60353=CARTESIAN_POINT('',(-24.48,21.616,21.216));
#60354=CARTESIAN_POINT('Origin',(-24.4189556308608,21.616,21.616));
#60355=CARTESIAN_POINT('',(-25.704,21.616,21.216));
#60356=CARTESIAN_POINT('Origin',(-30.3776010347741,21.616,23.4780766887229));
#60357=CARTESIAN_POINT('',(-37.3227504587735,21.216,25.6484358837227));
#60358=CARTESIAN_POINT('',(-30.3776010347741,21.216,23.4780766887229));
#60359=CARTESIAN_POINT('',(-37.536,21.616,25.296));
#60360=CARTESIAN_POINT('Origin',(-37.3227504587735,21.616,25.6484358837227));
#60361=CARTESIAN_POINT('',(-30.4969110320285,21.616,23.0962846975089));
#60362=CARTESIAN_POINT('Origin',(-38.964,21.616,43.664));
#60363=CARTESIAN_POINT('',(-37.536,21.616,44.064));
#60364=CARTESIAN_POINT('',(-44.064,21.616,44.064));
#60365=CARTESIAN_POINT('',(-38.964,21.616,44.064));
#60366=CARTESIAN_POINT('',(-44.064,21.216,43.664));
#60367=CARTESIAN_POINT('Origin',(-44.064,21.616,43.664));
#60368=CARTESIAN_POINT('',(-37.4710889359326,21.216,43.664));
#60369=CARTESIAN_POINT('',(-38.964,21.216,43.664));
#60370=CARTESIAN_POINT('Origin',(-37.4710889359326,21.616,43.664));
#60371=CARTESIAN_POINT('Origin',(-37.3483088935933,21.616,43.7049266807798));
#60372=CARTESIAN_POINT('',(-32.5750889359327,21.216,45.296));
#60373=CARTESIAN_POINT('',(-37.3483088935933,21.216,43.7049266807798));
#60374=CARTESIAN_POINT('Origin',(-32.5750889359327,21.616,45.296));
#60375=CARTESIAN_POINT('',(-37.4748,21.616,44.0844));
#60376=CARTESIAN_POINT('Origin',(-18.368,1.624,45.296));
#60377=CARTESIAN_POINT('Origin',(-18.368,1.624,45.296));
#60378=CARTESIAN_POINT('',(-18.368,1.224,45.296));
#60379=CARTESIAN_POINT('Origin',(-18.368,1.624,45.296));
#60380=CARTESIAN_POINT('Origin',(-18.368,1.624,45.296));
#60381=CARTESIAN_POINT('Origin',(-18.368,1.224,45.296));
#60382=CARTESIAN_POINT('Origin',(-18.368,21.616,45.296));
#60383=CARTESIAN_POINT('Origin',(-26.316,21.616,45.296));
#60384=CARTESIAN_POINT('',(-26.316,21.216,45.296));
#60385=CARTESIAN_POINT('Origin',(-44.064,21.616,37.944));
#60386=CARTESIAN_POINT('',(-43.9006475697477,21.216,32.226332994697));
#60387=CARTESIAN_POINT('Origin',(-44.064,21.216,37.944));
#60388=CARTESIAN_POINT('',(-44.064,21.616,31.824));
#60389=CARTESIAN_POINT('Origin',(-44.064,21.616,37.944));
#60390=CARTESIAN_POINT('Ctrl Pts',(-44.064,21.616,31.824));
#60391=CARTESIAN_POINT('Ctrl Pts',(-44.064,21.5840682080023,31.824));
#60392=CARTESIAN_POINT('Ctrl Pts',(-44.0624149120547,21.5524184382745,31.8278216249186));
#60393=CARTESIAN_POINT('Ctrl Pts',(-44.0593318094221,21.5217063486302,31.8352741901928));
#60394=CARTESIAN_POINT('Ctrl Pts',(-44.0577471400151,21.5059207862653,31.8391046991316));
#60395=CARTESIAN_POINT('Ctrl Pts',(-44.0557666149525,21.4903819028471,31.843894541907));
#60396=CARTESIAN_POINT('Ctrl Pts',(-44.0534015865836,21.475175853192,31.8496182972997));
#60397=CARTESIAN_POINT('Ctrl Pts',(-44.0495756131013,21.4505765953079,31.8588777787669));
#60398=CARTESIAN_POINT('Ctrl Pts',(-44.0447927695183,21.4271697387686,31.8704588320918));
#60399=CARTESIAN_POINT('Ctrl Pts',(-44.0391810250039,21.4052271621859,31.8840862281474));
#60400=CARTESIAN_POINT('Ctrl Pts',(-44.0341776804514,21.3856635005241,31.8962362035505));
#60401=CARTESIAN_POINT('Ctrl Pts',(-44.0285149435481,21.3672620257947,31.9100133437439));
#60402=CARTESIAN_POINT('Ctrl Pts',(-44.0222720478219,21.3501947099065,31.9252340460289));
#60403=CARTESIAN_POINT('Ctrl Pts',(-44.0152384316176,21.3309656606226,31.9423825910193));
#60404=CARTESIAN_POINT('Ctrl Pts',(-44.0075357743028,21.3136149870718,31.9611976208913));
#60405=CARTESIAN_POINT('Ctrl Pts',(-43.9993191486927,21.2982764025804,31.9813427758152));
#60406=CARTESIAN_POINT('Ctrl Pts',(-43.990799466837,21.2823720805162,32.0022309504784));
#60407=CARTESIAN_POINT('Ctrl Pts',(-43.9817264778667,21.2686293158374,32.0245499043989));
#60408=CARTESIAN_POINT('Ctrl Pts',(-43.9722455966321,21.2571751454754,32.0479521273707));
#60409=CARTESIAN_POINT('Ctrl Pts',(-43.9611780430457,21.2438040630693,32.0752708280667));
#60410=CARTESIAN_POINT('Ctrl Pts',(-43.9496295400104,21.233637777512,32.1038928160359));
#60411=CARTESIAN_POINT('Ctrl Pts',(-43.9378427069995,21.2267529507217,32.1332458643287));
#60412=CARTESIAN_POINT('Ctrl Pts',(-43.9259526178902,21.2198078108386,32.1628560538942));
#60413=CARTESIAN_POINT('Ctrl Pts',(-43.9138558645576,21.2162224659953,32.1931211104425));
#60414=CARTESIAN_POINT('Ctrl Pts',(-43.9017875351294,21.21601003407,32.2234661770043));
#60415=CARTESIAN_POINT('Ctrl Pts',(-43.9014075008992,21.216003344544,32.2244217495283));
#60416=CARTESIAN_POINT('Ctrl Pts',(-43.9010275100446,21.216,32.2253773614068));
#60417=CARTESIAN_POINT('Ctrl Pts',(-43.9006475697477,21.216,32.226332994697));
#60418=CARTESIAN_POINT('Origin',(-38.3751572875254,21.616,26.7008427124746));
#60419=CARTESIAN_POINT('',(-38.3751572875254,21.216,26.7008427124746));
#60420=CARTESIAN_POINT('',(-38.658,21.616,26.418));
#60421=CARTESIAN_POINT('Origin',(-17.544,21.216,21.216));
#60422=CARTESIAN_POINT('',(-24.48,22.04,21.216));
#60423=CARTESIAN_POINT('',(-24.48,21.216,21.216));
#60424=CARTESIAN_POINT('',(-25.704,22.04,21.216));
#60425=CARTESIAN_POINT('Origin',(-24.48,21.216,21.216));
#60426=CARTESIAN_POINT('',(-37.536,22.04,25.296));
#60427=CARTESIAN_POINT('',(-37.536,21.216,25.296));
#60428=CARTESIAN_POINT('',(-30.4969110320285,22.04,23.0962846975089));
#60429=CARTESIAN_POINT('Origin',(-37.536,21.216,25.296));
#60430=CARTESIAN_POINT('',(-44.064,22.04,31.824));
#60431=CARTESIAN_POINT('',(-44.064,21.216,31.824));
#60432=CARTESIAN_POINT('',(-38.658,22.04,26.418));
#60433=CARTESIAN_POINT('Origin',(-44.064,21.216,37.944));
#60434=CARTESIAN_POINT('',(-44.064,22.04,44.064));
#60435=CARTESIAN_POINT('',(-44.064,21.216,44.064));
#60436=CARTESIAN_POINT('Origin',(-44.064,22.04,37.944));
#60437=CARTESIAN_POINT('Origin',(-44.064,21.216,44.064));
#60438=CARTESIAN_POINT('',(-37.536,22.04,44.064));
#60439=CARTESIAN_POINT('',(-37.536,21.216,44.064));
#60440=CARTESIAN_POINT('',(-38.964,22.04,44.064));
#60441=CARTESIAN_POINT('Origin',(-37.536,21.216,44.064));
#60442=CARTESIAN_POINT('',(-37.4748,22.04,44.0844));
#60443=CARTESIAN_POINT('Origin',(-9.384,1.624,45.296));
#60444=CARTESIAN_POINT('',(-9.384,1.224,45.296));
#60445=CARTESIAN_POINT('Origin',(-18.368,1.624,37.74));
#60446=CARTESIAN_POINT('',(-18.368,1.224,36.0696854249492));
#60447=CARTESIAN_POINT('Origin',(-18.368,1.624,36.0696854249492));
#60448=CARTESIAN_POINT('',(-18.368,1.224,37.74));
#60449=CARTESIAN_POINT('Origin',(17.944,6.528,45.296));
#60450=CARTESIAN_POINT('',(17.544,2.448,45.296));
#60451=CARTESIAN_POINT('Origin',(17.944,2.048,45.296));
#60452=CARTESIAN_POINT('',(17.544,22.04,45.296));
#60453=CARTESIAN_POINT('Origin',(17.944,22.04,45.296));
#60454=CARTESIAN_POINT('',(17.544,6.528,45.296));
#60455=CARTESIAN_POINT('Origin',(17.944,22.04,45.296));
#60456=CARTESIAN_POINT('',(17.944,22.44,45.296));
#60457=CARTESIAN_POINT('Origin',(17.944,22.04,45.296));
#60458=CARTESIAN_POINT('Origin',(17.944,22.04,45.296));
#60459=CARTESIAN_POINT('Origin',(7.548,22.04,45.296));
#60460=CARTESIAN_POINT('',(32.5750889359327,22.44,45.296));
#60461=CARTESIAN_POINT('Origin',(32.5750889359327,22.04,45.296));
#60462=CARTESIAN_POINT('',(7.548,22.44,45.296));
#60463=CARTESIAN_POINT('Origin',(17.944,6.79529610292802,35.5539525918361));
#60464=CARTESIAN_POINT('',(17.544,21.616,32.9764388706062));
#60465=CARTESIAN_POINT('Origin',(17.944,21.616,32.9764388706062));
#60466=CARTESIAN_POINT('',(17.544,2.448,36.3100040879975));
#60467=CARTESIAN_POINT('Origin',(17.944,2.448,36.3100040879975));
#60468=CARTESIAN_POINT('',(17.544,6.79529610292802,35.5539525918361));
#60469=CARTESIAN_POINT('Origin',(17.944,10.404,38.36));
#60470=CARTESIAN_POINT('',(17.544,14.272,38.36));
#60471=CARTESIAN_POINT('',(17.544,8.576,38.36));
#60472=CARTESIAN_POINT('',(17.544,10.404,38.36));
#60473=CARTESIAN_POINT('',(17.944,8.976,38.76));
#60474=CARTESIAN_POINT('Origin',(17.944,8.576,38.36));
#60475=CARTESIAN_POINT('',(17.944,10.404,38.76));
#60476=CARTESIAN_POINT('Origin',(17.944,14.272,38.36));
#60477=CARTESIAN_POINT('Origin',(17.944,12.852,42.016));
#60478=CARTESIAN_POINT('',(17.544,8.576,42.016));
#60479=CARTESIAN_POINT('',(17.544,14.272,42.016));
#60480=CARTESIAN_POINT('',(17.544,12.852,42.016));
#60481=CARTESIAN_POINT('Origin',(17.944,14.272,42.016));
#60482=CARTESIAN_POINT('Origin',(17.944,8.576,42.016));
#60483=CARTESIAN_POINT('Origin',(17.944,14.272,38.964));
#60484=CARTESIAN_POINT('',(17.544,14.272,38.964));
#60485=CARTESIAN_POINT('Origin',(17.944,8.576,40.392));
#60486=CARTESIAN_POINT('',(17.544,8.576,40.392));
#60487=CARTESIAN_POINT('',(17.944,8.976,40.392));
#60488=CARTESIAN_POINT('Origin',(17.544,8.976,41.616));
#60489=CARTESIAN_POINT('',(17.544,8.976,38.76));
#60490=CARTESIAN_POINT('Origin',(17.544,11.832,39.168));
#60491=CARTESIAN_POINT('',(17.544,22.04,21.216));
#60492=CARTESIAN_POINT('',(17.544,22.04,36.312));
#60493=CARTESIAN_POINT('',(17.544,21.616,21.216));
#60494=CARTESIAN_POINT('',(17.544,21.216,21.216));
#60495=CARTESIAN_POINT('',(17.544,21.616,36.312));
#60496=CARTESIAN_POINT('',(17.544,2.448,39.372));
#60497=CARTESIAN_POINT('Origin',(35.7,21.616,43.664));
#60498=CARTESIAN_POINT('',(44.064,21.216,43.664));
#60499=CARTESIAN_POINT('',(44.064,21.616,44.064));
#60500=CARTESIAN_POINT('Origin',(44.064,21.616,43.664));
#60501=CARTESIAN_POINT('',(35.7,21.616,44.064));
#60502=CARTESIAN_POINT('',(35.7,21.216,43.664));
#60503=CARTESIAN_POINT('Origin',(44.064,21.616,37.944));
#60504=CARTESIAN_POINT('',(44.064,21.616,31.824));
#60505=CARTESIAN_POINT('Origin',(44.064,21.616,37.944));
#60506=CARTESIAN_POINT('',(43.9006475697477,21.216,32.226332994697));
#60507=CARTESIAN_POINT('Origin',(44.064,21.216,37.944));
#60508=CARTESIAN_POINT('Ctrl Pts',(43.9006475697477,21.216,32.226332994697));
#60509=CARTESIAN_POINT('Ctrl Pts',(43.9010275100447,21.216,32.2253773614065));
#60510=CARTESIAN_POINT('Ctrl Pts',(43.901407500899,21.216003344544,32.2244217495286));
#60511=CARTESIAN_POINT('Ctrl Pts',(43.9017875351293,21.21601003407,32.2234661770043));
#60512=CARTESIAN_POINT('Ctrl Pts',(43.9138558645572,21.2162224659953,32.193121110443));
#60513=CARTESIAN_POINT('Ctrl Pts',(43.9259526178902,21.2198078108386,32.1628560538943));
#60514=CARTESIAN_POINT('Ctrl Pts',(43.9378427069995,21.2267529507217,32.1332458643287));
#60515=CARTESIAN_POINT('Ctrl Pts',(43.9496295400104,21.233637777512,32.1038928160359));
#60516=CARTESIAN_POINT('Ctrl Pts',(43.9611780430457,21.2438040630693,32.0752708280668));
#60517=CARTESIAN_POINT('Ctrl Pts',(43.9722455966321,21.2571751454754,32.0479521273707));
#60518=CARTESIAN_POINT('Ctrl Pts',(43.9820721961623,21.2690469896968,32.0236965473702));
#60519=CARTESIAN_POINT('Ctrl Pts',(43.9914607629778,21.2833774561247,32.0006045298454));
#60520=CARTESIAN_POINT('Ctrl Pts',(44.0002489315777,21.300024857828,31.9790634597097));
#60521=CARTESIAN_POINT('Ctrl Pts',(44.0081171229227,21.3149295493471,31.9597773866584));
#60522=CARTESIAN_POINT('Ctrl Pts',(44.0155043707225,21.3316927057167,31.9417342092235));
#60523=CARTESIAN_POINT('Ctrl Pts',(44.0222720478219,21.3501947099065,31.9252340460289));
#60524=CARTESIAN_POINT('Ctrl Pts',(44.029760827937,21.3706681218367,31.9069757733286));
#60525=CARTESIAN_POINT('Ctrl Pts',(44.0364152831142,21.393062029884,31.8907942319792));
#60526=CARTESIAN_POINT('Ctrl Pts',(44.0420970014355,21.4170773367871,31.8770079892748));
#60527=CARTESIAN_POINT('Ctrl Pts',(44.0464641694145,21.4355363439712,31.8664113996019));
#60528=CARTESIAN_POINT('Ctrl Pts',(44.0502563764082,21.4549535917043,31.8572302202428));
#60529=CARTESIAN_POINT('Ctrl Pts',(44.0534015865836,21.475175853192,31.8496182972998));
#60530=CARTESIAN_POINT('Ctrl Pts',(44.0584453970152,21.5076052451096,31.8374114512694));
#60531=CARTESIAN_POINT('Ctrl Pts',(44.0617407660415,21.5415499503757,31.8294519002684));
#60532=CARTESIAN_POINT('Ctrl Pts',(44.0631761028331,21.57616875624,31.8259877017421));
#60533=CARTESIAN_POINT('Ctrl Pts',(44.0637232166716,21.5893645635749,31.824667237469));
#60534=CARTESIAN_POINT('Ctrl Pts',(44.064,21.6026580205647,31.824));
#60535=CARTESIAN_POINT('Ctrl Pts',(44.064,21.616,31.824));
#60536=CARTESIAN_POINT('Origin',(41.6391572875254,21.616,29.9648427124746));
#60537=CARTESIAN_POINT('',(37.3227504587735,21.216,25.6484358837227));
#60538=CARTESIAN_POINT('',(41.6391572875254,21.216,29.9648427124746));
#60539=CARTESIAN_POINT('',(37.536,21.616,25.296));
#60540=CARTESIAN_POINT('Origin',(37.3227504587735,21.616,25.6484358837227));
#60541=CARTESIAN_POINT('',(41.922,21.616,29.682));
#60542=CARTESIAN_POINT('Origin',(36.9056010347741,21.616,25.5180766887229));
#60543=CARTESIAN_POINT('',(24.4189556308608,21.216,21.616));
#60544=CARTESIAN_POINT('',(36.9056010347741,21.216,25.5180766887229));
#60545=CARTESIAN_POINT('',(24.48,21.616,21.216));
#60546=CARTESIAN_POINT('Origin',(24.4189556308608,21.616,21.616));
#60547=CARTESIAN_POINT('',(37.0249110320285,21.616,25.1362846975089));
#60548=CARTESIAN_POINT('Origin',(17.944,21.616,36.312));
#60549=CARTESIAN_POINT('',(17.944,21.216,21.616));
#60550=CARTESIAN_POINT('',(17.944,21.216,36.312));
#60551=CARTESIAN_POINT('Origin',(17.944,21.616,21.616));
#60552=CARTESIAN_POINT('Origin',(29.172,21.616,21.616));
#60553=CARTESIAN_POINT('',(29.172,21.216,21.616));
#60554=CARTESIAN_POINT('',(29.172,21.616,21.216));
#60555=CARTESIAN_POINT('Origin',(37.536,21.216,44.064));
#60556=CARTESIAN_POINT('',(44.064,22.04,44.064));
#60557=CARTESIAN_POINT('',(44.064,21.216,44.064));
#60558=CARTESIAN_POINT('',(35.7,22.04,44.064));
#60559=CARTESIAN_POINT('Origin',(44.064,21.216,37.944));
#60560=CARTESIAN_POINT('',(44.064,22.04,31.824));
#60561=CARTESIAN_POINT('',(44.064,21.216,31.824));
#60562=CARTESIAN_POINT('Origin',(44.064,22.04,37.944));
#60563=CARTESIAN_POINT('Origin',(44.064,21.216,31.824));
#60564=CARTESIAN_POINT('',(37.536,22.04,25.296));
#60565=CARTESIAN_POINT('',(37.536,21.216,25.296));
#60566=CARTESIAN_POINT('',(41.922,22.04,29.682));
#60567=CARTESIAN_POINT('Origin',(37.536,21.216,25.296));
#60568=CARTESIAN_POINT('',(24.48,22.04,21.216));
#60569=CARTESIAN_POINT('',(24.48,21.216,21.216));
#60570=CARTESIAN_POINT('',(37.0249110320285,22.04,25.1362846975089));
#60571=CARTESIAN_POINT('Origin',(24.48,21.216,21.216));
#60572=CARTESIAN_POINT('',(29.172,22.04,21.216));
#60573=CARTESIAN_POINT('Origin',(-37.3483088935933,22.04,43.7049266807798));
#60574=CARTESIAN_POINT('',(-37.4710889359326,22.44,43.664));
#60575=CARTESIAN_POINT('',(-37.3483088935933,22.44,43.7049266807798));
#60576=CARTESIAN_POINT('Origin',(-37.4710889359326,22.04,43.664));
#60577=CARTESIAN_POINT('Origin',(-44.064,22.04,37.944));
#60578=CARTESIAN_POINT('',(-44.064,22.44,43.664));
#60579=CARTESIAN_POINT('Origin',(-44.064,22.04,43.664));
#60580=CARTESIAN_POINT('',(-43.9006475697477,22.44,32.226332994697));
#60581=CARTESIAN_POINT('Origin',(-44.064,22.44,37.944));
#60582=CARTESIAN_POINT('Ctrl Pts',(-43.9006475697477,22.44,32.226332994697));
#60583=CARTESIAN_POINT('Ctrl Pts',(-43.901027510044,22.44,32.2253773614083));
#60584=CARTESIAN_POINT('Ctrl Pts',(-43.9014075009006,22.439996655456,32.2244217495276));
#60585=CARTESIAN_POINT('Ctrl Pts',(-43.90178753513,22.43998996593,32.223466177005));
#60586=CARTESIAN_POINT('Ctrl Pts',(-43.9138558645418,22.4397775340048,32.1931211104619));
#60587=CARTESIAN_POINT('Ctrl Pts',(-43.9259526178886,22.4361921891623,32.1628560538983));
#60588=CARTESIAN_POINT('Ctrl Pts',(-43.9378427069994,22.4292470492784,32.133245864329));
#60589=CARTESIAN_POINT('Ctrl Pts',(-43.9496295400103,22.4223622224881,32.1038928160361));
#60590=CARTESIAN_POINT('Ctrl Pts',(-43.9611780430457,22.4121959369308,32.0752708280669));
#60591=CARTESIAN_POINT('Ctrl Pts',(-43.9722455966321,22.3988248545246,32.0479521273707));
#60592=CARTESIAN_POINT('Ctrl Pts',(-43.9820721961623,22.3869530103033,32.0236965473703));
#60593=CARTESIAN_POINT('Ctrl Pts',(-43.9914607629777,22.3726225438754,32.0006045298457));
#60594=CARTESIAN_POINT('Ctrl Pts',(-44.0002489315775,22.3559751421723,31.9790634597102));
#60595=CARTESIAN_POINT('Ctrl Pts',(-44.0081171229226,22.3410704506531,31.9597773866587));
#60596=CARTESIAN_POINT('Ctrl Pts',(-44.0155043707224,22.3243072942834,31.9417342092236));
#60597=CARTESIAN_POINT('Ctrl Pts',(-44.0222720478219,22.3058052900935,31.9252340460289));
#60598=CARTESIAN_POINT('Ctrl Pts',(-44.0297608279369,22.2853318781636,31.9069757733289));
#60599=CARTESIAN_POINT('Ctrl Pts',(-44.036415283114,22.2629379701166,31.8907942319796));
#60600=CARTESIAN_POINT('Ctrl Pts',(-44.0420970014353,22.238922663214,31.8770079892754));
#60601=CARTESIAN_POINT('Ctrl Pts',(-44.0464641694143,22.2204636560296,31.8664113996022));
#60602=CARTESIAN_POINT('Ctrl Pts',(-44.0502563764081,22.2010464082961,31.8572302202429));
#60603=CARTESIAN_POINT('Ctrl Pts',(-44.0534015865836,22.180824146808,31.8496182972997));
#60604=CARTESIAN_POINT('Ctrl Pts',(-44.0584453970151,22.1483947548905,31.8374114512694));
#60605=CARTESIAN_POINT('Ctrl Pts',(-44.0617407660415,22.1144500496243,31.8294519002684));
#60606=CARTESIAN_POINT('Ctrl Pts',(-44.063176102833,22.0798312437601,31.8259877017421));
#60607=CARTESIAN_POINT('Ctrl Pts',(-44.0637232166716,22.0666354364251,31.824667237469));
#60608=CARTESIAN_POINT('Ctrl Pts',(-44.064,22.0533419794354,31.824));
#60609=CARTESIAN_POINT('Ctrl Pts',(-44.064,22.04,31.824));
#60610=CARTESIAN_POINT('Origin',(-38.964,22.04,43.664));
#60611=CARTESIAN_POINT('',(-38.964,22.44,43.664));
#60612=CARTESIAN_POINT('Origin',(-38.3751572875254,22.04,26.7008427124746));
#60613=CARTESIAN_POINT('',(-37.3227504587735,22.44,25.6484358837227));
#60614=CARTESIAN_POINT('',(-38.3751572875254,22.44,26.7008427124746));
#60615=CARTESIAN_POINT('Origin',(-37.3227504587735,22.04,25.6484358837227));
#60616=CARTESIAN_POINT('Origin',(-30.3776010347741,22.04,23.4780766887229));
#60617=CARTESIAN_POINT('',(-24.4189556308608,22.44,21.616));
#60618=CARTESIAN_POINT('',(-30.3776010347741,22.44,23.4780766887229));
#60619=CARTESIAN_POINT('Origin',(-24.4189556308608,22.04,21.616));
#60620=CARTESIAN_POINT('Origin',(-25.704,22.04,21.616));
#60621=CARTESIAN_POINT('',(-25.704,22.44,21.616));
#60622=CARTESIAN_POINT('Origin',(-33.864,22.44,33.456));
#60623=CARTESIAN_POINT('',(-29.376,22.44,42.424));
#60624=CARTESIAN_POINT('Origin',(-29.376,22.44,38.352));
#60625=CARTESIAN_POINT('',(-44.064,22.44,40.792));
#60626=CARTESIAN_POINT('Origin',(-44.064,22.44,37.944));
#60627=CARTESIAN_POINT('',(-28.152,22.44,31.46));
#60628=CARTESIAN_POINT('Origin',(-28.152,22.44,28.56));
#60629=CARTESIAN_POINT('Origin',(-29.376,21.1264,38.352));
#60630=CARTESIAN_POINT('',(-29.376,20.7264,44.072));
#60631=CARTESIAN_POINT('Origin',(-29.376,20.7264,38.352));
#60632=CARTESIAN_POINT('',(-29.376,21.1264,44.472));
#60633=CARTESIAN_POINT('Origin',(-29.376,21.1264,44.072));
#60634=CARTESIAN_POINT('',(-35.496,21.1264,38.352));
#60635=CARTESIAN_POINT('Origin',(-29.376,21.1264,38.352));
#60636=CARTESIAN_POINT('Origin',(-29.376,21.1264,38.352));
#60637=CARTESIAN_POINT('Origin',(-29.376,20.7264,38.352));
#60638=CARTESIAN_POINT('',(-29.376,20.7264,34.28));
#60639=CARTESIAN_POINT('Origin',(-29.376,20.7264,38.352));
#60640=CARTESIAN_POINT('Origin',(-29.376,21.216,38.352));
#60641=CARTESIAN_POINT('',(-35.496,21.216,38.352));
#60642=CARTESIAN_POINT('',(-35.496,21.216,38.352));
#60643=CARTESIAN_POINT('Origin',(-29.376,21.216,38.352));
#60644=CARTESIAN_POINT('Origin',(35.7,22.04,43.664));
#60645=CARTESIAN_POINT('',(44.064,22.44,43.664));
#60646=CARTESIAN_POINT('Origin',(44.064,22.04,43.664));
#60647=CARTESIAN_POINT('',(37.4710889359326,22.44,43.664));
#60648=CARTESIAN_POINT('',(35.7,22.44,43.664));
#60649=CARTESIAN_POINT('Origin',(37.4710889359326,22.04,43.664));
#60650=CARTESIAN_POINT('Origin',(34.9003088935933,22.04,44.5209266807798));
#60651=CARTESIAN_POINT('',(34.9003088935933,22.44,44.5209266807798));
#60652=CARTESIAN_POINT('Origin',(17.944,22.04,36.312));
#60653=CARTESIAN_POINT('',(17.944,22.44,21.616));
#60654=CARTESIAN_POINT('',(17.944,22.44,36.312));
#60655=CARTESIAN_POINT('Origin',(17.944,22.04,21.616));
#60656=CARTESIAN_POINT('Origin',(29.172,22.04,21.616));
#60657=CARTESIAN_POINT('',(24.4189556308608,22.44,21.616));
#60658=CARTESIAN_POINT('',(29.172,22.44,21.616));
#60659=CARTESIAN_POINT('Origin',(24.4189556308608,22.04,21.616));
#60660=CARTESIAN_POINT('Origin',(36.9056010347741,22.04,25.5180766887229));
#60661=CARTESIAN_POINT('',(37.3227504587735,22.44,25.6484358837227));
#60662=CARTESIAN_POINT('',(36.9056010347741,22.44,25.5180766887229));
#60663=CARTESIAN_POINT('Origin',(37.3227504587735,22.04,25.6484358837227));
#60664=CARTESIAN_POINT('Origin',(41.6391572875254,22.04,29.9648427124746));
#60665=CARTESIAN_POINT('',(43.9006475697477,22.44,32.226332994697));
#60666=CARTESIAN_POINT('',(41.6391572875254,22.44,29.9648427124746));
#60667=CARTESIAN_POINT('Ctrl Pts',(43.9006475697477,22.44,32.226332994697));
#60668=CARTESIAN_POINT('Ctrl Pts',(43.9010275100447,22.44,32.2253773614065));
#60669=CARTESIAN_POINT('Ctrl Pts',(43.901407500899,22.439996655456,32.2244217495286));
#60670=CARTESIAN_POINT('Ctrl Pts',(43.9017875351293,22.43998996593,32.2234661770043));
#60671=CARTESIAN_POINT('Ctrl Pts',(43.9138558645572,22.4397775340047,32.193121110443));
#60672=CARTESIAN_POINT('Ctrl Pts',(43.9259526178902,22.4361921891614,32.1628560538943));
#60673=CARTESIAN_POINT('Ctrl Pts',(43.9378427069995,22.4292470492783,32.1332458643287));
#60674=CARTESIAN_POINT('Ctrl Pts',(43.9496295400103,22.422362222488,32.103892816036));
#60675=CARTESIAN_POINT('Ctrl Pts',(43.9611780430457,22.4121959369307,32.0752708280668));
#60676=CARTESIAN_POINT('Ctrl Pts',(43.9722455966321,22.3988248545246,32.0479521273707));
#60677=CARTESIAN_POINT('Ctrl Pts',(43.9820721961622,22.3869530103033,32.0236965473703));
#60678=CARTESIAN_POINT('Ctrl Pts',(43.9914607629777,22.3726225438755,32.0006045298457));
#60679=CARTESIAN_POINT('Ctrl Pts',(44.0002489315775,22.3559751421724,31.9790634597103));
#60680=CARTESIAN_POINT('Ctrl Pts',(44.0081171229226,22.3410704506532,31.9597773866587));
#60681=CARTESIAN_POINT('Ctrl Pts',(44.0155043707224,22.3243072942834,31.9417342092237));
#60682=CARTESIAN_POINT('Ctrl Pts',(44.0222720478219,22.3058052900935,31.9252340460289));
#60683=CARTESIAN_POINT('Ctrl Pts',(44.029760827937,22.2853318781633,31.9069757733286));
#60684=CARTESIAN_POINT('Ctrl Pts',(44.0364152831142,22.262937970116,31.8907942319792));
#60685=CARTESIAN_POINT('Ctrl Pts',(44.0420970014355,22.2389226632129,31.8770079892748));
#60686=CARTESIAN_POINT('Ctrl Pts',(44.0464641694145,22.2204636560288,31.8664113996019));
#60687=CARTESIAN_POINT('Ctrl Pts',(44.0502563764082,22.2010464082957,31.8572302202428));
#60688=CARTESIAN_POINT('Ctrl Pts',(44.0534015865836,22.180824146808,31.8496182972998));
#60689=CARTESIAN_POINT('Ctrl Pts',(44.0584453970152,22.1483947548904,31.8374114512694));
#60690=CARTESIAN_POINT('Ctrl Pts',(44.0617407660415,22.1144500496243,31.8294519002684));
#60691=CARTESIAN_POINT('Ctrl Pts',(44.0631761028331,22.07983124376,31.8259877017421));
#60692=CARTESIAN_POINT('Ctrl Pts',(44.0637232166716,22.0666354364251,31.824667237469));
#60693=CARTESIAN_POINT('Ctrl Pts',(44.064,22.0533419794353,31.824));
#60694=CARTESIAN_POINT('Ctrl Pts',(44.064,22.04,31.824));
#60695=CARTESIAN_POINT('Origin',(44.064,22.04,37.944));
#60696=CARTESIAN_POINT('Origin',(44.064,22.44,37.944));
#60697=CARTESIAN_POINT('Origin',(33.864,22.44,33.456));
#60698=CARTESIAN_POINT('',(29.376,22.44,42.424));
#60699=CARTESIAN_POINT('Origin',(29.376,22.44,38.352));
#60700=CARTESIAN_POINT('',(28.152,22.44,31.46));
#60701=CARTESIAN_POINT('Origin',(28.152,22.44,28.56));
#60702=CARTESIAN_POINT('',(44.064,22.44,40.792));
#60703=CARTESIAN_POINT('Origin',(44.064,22.44,37.944));
#60704=CARTESIAN_POINT('Origin',(29.376,21.1264,38.352));
#60705=CARTESIAN_POINT('',(29.376,20.7264,44.072));
#60706=CARTESIAN_POINT('Origin',(29.376,20.7264,38.352));
#60707=CARTESIAN_POINT('',(29.376,21.1264,44.472));
#60708=CARTESIAN_POINT('Origin',(29.376,21.1264,44.072));
#60709=CARTESIAN_POINT('',(23.256,21.1264,38.352));
#60710=CARTESIAN_POINT('Origin',(29.376,21.1264,38.352));
#60711=CARTESIAN_POINT('Origin',(29.376,21.1264,38.352));
#60712=CARTESIAN_POINT('Origin',(29.376,20.7264,38.352));
#60713=CARTESIAN_POINT('',(29.376,20.7264,34.28));
#60714=CARTESIAN_POINT('Origin',(29.376,20.7264,38.352));
#60715=CARTESIAN_POINT('Origin',(29.376,21.216,38.352));
#60716=CARTESIAN_POINT('',(23.256,21.216,38.352));
#60717=CARTESIAN_POINT('',(23.256,21.216,38.352));
#60718=CARTESIAN_POINT('Origin',(29.376,21.216,38.352));
#60719=CARTESIAN_POINT('Origin',(29.376,21.1264,38.352));
#60720=CARTESIAN_POINT('',(29.376,21.1264,34.68));
#60721=CARTESIAN_POINT('Origin',(29.376,21.1264,34.28));
#60722=CARTESIAN_POINT('',(25.704,21.1264,38.352));
#60723=CARTESIAN_POINT('Origin',(29.376,21.1264,38.352));
#60724=CARTESIAN_POINT('Origin',(29.376,21.1264,38.352));
#60725=CARTESIAN_POINT('Origin',(29.376,20.7264,38.352));
#60726=CARTESIAN_POINT('',(25.704,22.04,38.352));
#60727=CARTESIAN_POINT('',(25.704,20.7264,38.352));
#60728=CARTESIAN_POINT('',(29.376,22.04,42.024));
#60729=CARTESIAN_POINT('Origin',(29.376,22.04,38.352));
#60730=CARTESIAN_POINT('Origin',(29.376,22.04,38.352));
#60731=CARTESIAN_POINT('Origin',(29.376,22.04,38.352));
#60732=CARTESIAN_POINT('Origin',(29.376,22.04,42.424));
#60733=CARTESIAN_POINT('Origin',(-29.376,21.1264,38.352));
#60734=CARTESIAN_POINT('',(-29.376,21.1264,34.68));
#60735=CARTESIAN_POINT('Origin',(-29.376,21.1264,34.28));
#60736=CARTESIAN_POINT('',(-33.048,21.1264,38.352));
#60737=CARTESIAN_POINT('Origin',(-29.376,21.1264,38.352));
#60738=CARTESIAN_POINT('Origin',(-29.376,21.1264,38.352));
#60739=CARTESIAN_POINT('Origin',(-29.376,20.7264,38.352));
#60740=CARTESIAN_POINT('',(-33.048,22.04,38.352));
#60741=CARTESIAN_POINT('',(-33.048,20.7264,38.352));
#60742=CARTESIAN_POINT('',(-29.376,22.04,42.024));
#60743=CARTESIAN_POINT('Origin',(-29.376,22.04,38.352));
#60744=CARTESIAN_POINT('Origin',(-29.376,22.04,38.352));
#60745=CARTESIAN_POINT('Origin',(-29.376,22.04,38.352));
#60746=CARTESIAN_POINT('Origin',(-29.376,22.04,42.424));
#60747=CARTESIAN_POINT('Origin',(44.064,22.04,37.944));
#60748=CARTESIAN_POINT('',(44.064,22.04,40.392));
#60749=CARTESIAN_POINT('Origin',(44.064,22.04,40.792));
#60750=CARTESIAN_POINT('',(41.616,22.04,37.944));
#60751=CARTESIAN_POINT('Origin',(44.064,22.04,37.944));
#60752=CARTESIAN_POINT('Origin',(44.064,22.04,37.944));
#60753=CARTESIAN_POINT('Origin',(44.064,20.7264,37.944));
#60754=CARTESIAN_POINT('',(44.064,21.616,35.496));
#60755=CARTESIAN_POINT('',(41.616,21.616,37.944));
#60756=CARTESIAN_POINT('Origin',(44.064,21.616,37.944));
#60757=CARTESIAN_POINT('Origin',(44.064,21.616,37.944));
#60758=CARTESIAN_POINT('',(41.616,20.7264,37.944));
#60759=CARTESIAN_POINT('Origin',(44.064,21.616,37.944));
#60760=CARTESIAN_POINT('',(44.064,21.216,35.096));
#60761=CARTESIAN_POINT('Origin',(44.064,21.216,37.944));
#60762=CARTESIAN_POINT('Origin',(44.064,21.616,35.096));
#60763=CARTESIAN_POINT('Origin',(33.864,21.216,33.456));
#60764=CARTESIAN_POINT('',(28.152,21.216,25.66));
#60765=CARTESIAN_POINT('Origin',(28.152,21.216,28.56));
#60766=CARTESIAN_POINT('Origin',(-28.152,22.04,28.56));
#60767=CARTESIAN_POINT('',(-28.152,22.04,31.06));
#60768=CARTESIAN_POINT('Origin',(-28.152,22.04,31.46));
#60769=CARTESIAN_POINT('',(-30.652,22.04,28.56));
#60770=CARTESIAN_POINT('Origin',(-28.152,22.04,28.56));
#60771=CARTESIAN_POINT('Origin',(-28.152,22.04,28.56));
#60772=CARTESIAN_POINT('Origin',(-28.152,20.7264,28.56));
#60773=CARTESIAN_POINT('',(-28.152,21.616,26.06));
#60774=CARTESIAN_POINT('',(-30.652,21.616,28.56));
#60775=CARTESIAN_POINT('Origin',(-28.152,21.616,28.56));
#60776=CARTESIAN_POINT('Origin',(-28.152,21.616,28.56));
#60777=CARTESIAN_POINT('',(-30.652,20.7264,28.56));
#60778=CARTESIAN_POINT('Origin',(-28.152,21.616,28.56));
#60779=CARTESIAN_POINT('',(-28.152,21.216,25.66));
#60780=CARTESIAN_POINT('Origin',(-28.152,21.216,28.56));
#60781=CARTESIAN_POINT('Origin',(-28.152,21.616,25.66));
#60782=CARTESIAN_POINT('Origin',(-33.864,21.216,33.456));
#60783=CARTESIAN_POINT('',(-17.544,21.216,32.64));
#60784=CARTESIAN_POINT('',(-44.064,21.216,35.096));
#60785=CARTESIAN_POINT('Origin',(-44.064,21.216,37.944));
#60786=CARTESIAN_POINT('Origin',(28.152,22.04,28.56));
#60787=CARTESIAN_POINT('',(28.152,22.04,31.06));
#60788=CARTESIAN_POINT('Origin',(28.152,22.04,31.46));
#60789=CARTESIAN_POINT('',(25.652,22.04,28.56));
#60790=CARTESIAN_POINT('Origin',(28.152,22.04,28.56));
#60791=CARTESIAN_POINT('Origin',(28.152,22.04,28.56));
#60792=CARTESIAN_POINT('Origin',(28.152,20.7264,28.56));
#60793=CARTESIAN_POINT('',(28.152,21.616,26.06));
#60794=CARTESIAN_POINT('',(25.652,21.616,28.56));
#60795=CARTESIAN_POINT('Origin',(28.152,21.616,28.56));
#60796=CARTESIAN_POINT('Origin',(28.152,21.616,28.56));
#60797=CARTESIAN_POINT('',(25.652,20.7264,28.56));
#60798=CARTESIAN_POINT('Origin',(28.152,21.616,28.56));
#60799=CARTESIAN_POINT('Origin',(28.152,21.616,25.66));
#60800=CARTESIAN_POINT('Origin',(-44.064,22.04,37.944));
#60801=CARTESIAN_POINT('',(-44.064,22.04,40.392));
#60802=CARTESIAN_POINT('Origin',(-44.064,22.04,40.792));
#60803=CARTESIAN_POINT('',(-46.512,22.04,37.944));
#60804=CARTESIAN_POINT('Origin',(-44.064,22.04,37.944));
#60805=CARTESIAN_POINT('Origin',(-44.064,22.04,37.944));
#60806=CARTESIAN_POINT('Origin',(-44.064,20.7264,37.944));
#60807=CARTESIAN_POINT('',(-44.064,21.616,35.496));
#60808=CARTESIAN_POINT('',(-46.512,21.616,37.944));
#60809=CARTESIAN_POINT('Origin',(-44.064,21.616,37.944));
#60810=CARTESIAN_POINT('Origin',(-44.064,21.616,37.944));
#60811=CARTESIAN_POINT('',(-46.512,20.7264,37.944));
#60812=CARTESIAN_POINT('Origin',(-44.064,21.616,37.944));
#60813=CARTESIAN_POINT('Origin',(-44.064,21.616,35.096));
#60814=CARTESIAN_POINT('Origin',(6.528,2.048,42.432));
#60815=CARTESIAN_POINT('',(6.528,2.448,44.132));
#60816=CARTESIAN_POINT('Origin',(6.528,2.448,42.432));
#60817=CARTESIAN_POINT('',(6.528,2.048,43.732));
#60818=CARTESIAN_POINT('Origin',(6.528,2.048,44.132));
#60819=CARTESIAN_POINT('',(5.228,2.048,42.432));
#60820=CARTESIAN_POINT('Origin',(6.528,2.048,42.432));
#60821=CARTESIAN_POINT('Origin',(6.528,2.048,42.432));
#60822=CARTESIAN_POINT('Origin',(6.528,1.224,42.432));
#60823=CARTESIAN_POINT('',(6.528,1.624,41.132));
#60824=CARTESIAN_POINT('',(5.228,1.624,42.432));
#60825=CARTESIAN_POINT('Origin',(6.528,1.624,42.432));
#60826=CARTESIAN_POINT('Origin',(6.528,1.624,42.432));
#60827=CARTESIAN_POINT('',(5.228,1.224,42.432));
#60828=CARTESIAN_POINT('Origin',(0.,2.448,39.576));
#60829=CARTESIAN_POINT('',(-18.2023145750508,2.448,35.904));
#60830=CARTESIAN_POINT('',(-16.1543145750508,2.448,33.856));
#60831=CARTESIAN_POINT('',(-13.4871572875254,2.448,31.1888427124746));
#60832=CARTESIAN_POINT('',(-8.772,2.448,35.904));
#60833=CARTESIAN_POINT('',(-9.384,2.448,45.296));
#60834=CARTESIAN_POINT('',(16.1543145750508,2.448,33.856));
#60835=CARTESIAN_POINT('',(14.7111572875254,2.448,32.4128427124746));
#60836=CARTESIAN_POINT('',(8.16,2.448,33.856));
#60837=CARTESIAN_POINT('',(-6.528,2.448,44.132));
#60838=CARTESIAN_POINT('Origin',(-6.528,2.448,42.432));
#60839=CARTESIAN_POINT('',(-15.904,2.448,35.504));
#60840=CARTESIAN_POINT('',(-15.904,2.448,41.608));
#60841=CARTESIAN_POINT('',(-15.904,2.448,37.74));
#60842=CARTESIAN_POINT('',(-12.656,2.448,35.504));
#60843=CARTESIAN_POINT('',(-6.528,2.448,35.504));
#60844=CARTESIAN_POINT('',(-12.656,2.448,41.608));
#60845=CARTESIAN_POINT('',(-12.656,2.448,40.392));
#60846=CARTESIAN_POINT('',(-7.752,2.448,41.608));
#60847=CARTESIAN_POINT('',(12.656,2.448,35.504));
#60848=CARTESIAN_POINT('',(12.656,2.448,41.608));
#60849=CARTESIAN_POINT('',(12.656,2.448,37.74));
#60850=CARTESIAN_POINT('',(15.904,2.448,35.504));
#60851=CARTESIAN_POINT('',(7.752,2.448,35.504));
#60852=CARTESIAN_POINT('',(15.904,2.448,41.608));
#60853=CARTESIAN_POINT('',(15.904,2.448,40.392));
#60854=CARTESIAN_POINT('',(6.528,2.448,41.608));
#60855=CARTESIAN_POINT('Origin',(-13.4871572875254,2.048,31.1888427124746));
#60856=CARTESIAN_POINT('',(-16.32,2.048,33.456));
#60857=CARTESIAN_POINT('',(-13.77,2.048,30.906));
#60858=CARTESIAN_POINT('Origin',(-18.2718797924421,2.048,35.9735652173913));
#60859=CARTESIAN_POINT('Origin',(-16.1543145750508,2.048,33.856));
#60860=CARTESIAN_POINT('Origin',(8.16,2.048,33.856));
#60861=CARTESIAN_POINT('',(16.32,2.048,33.456));
#60862=CARTESIAN_POINT('Origin',(16.1543145750508,2.048,33.856));
#60863=CARTESIAN_POINT('',(8.16,2.048,33.456));
#60864=CARTESIAN_POINT('Origin',(14.7111572875254,2.048,32.4128427124746));
#60865=CARTESIAN_POINT('',(14.994,2.048,32.13));
#60866=CARTESIAN_POINT('Origin',(-16.32,1.224,33.456));
#60867=CARTESIAN_POINT('',(-16.32,1.624,33.456));
#60868=CARTESIAN_POINT('',(-16.32,1.224,33.456));
#60869=CARTESIAN_POINT('',(-13.77,1.624,30.906));
#60870=CARTESIAN_POINT('Origin',(16.32,1.224,33.456));
#60871=CARTESIAN_POINT('',(16.32,1.624,33.456));
#60872=CARTESIAN_POINT('',(16.32,1.224,33.456));
#60873=CARTESIAN_POINT('',(8.16,1.624,33.456));
#60874=CARTESIAN_POINT('Origin',(18.768,1.224,35.904));
#60875=CARTESIAN_POINT('',(14.994,1.624,32.13));
#60876=CARTESIAN_POINT('Origin',(-9.384,2.048,45.296));
#60877=CARTESIAN_POINT('Origin',(6.528,1.624,42.432));
#60878=CARTESIAN_POINT('',(6.528,1.224,40.732));
#60879=CARTESIAN_POINT('Origin',(6.528,1.224,42.432));
#60880=CARTESIAN_POINT('Origin',(6.528,1.624,40.732));
#60881=CARTESIAN_POINT('Origin',(0.,1.224,39.576));
#60882=CARTESIAN_POINT('',(-16.1543145750508,1.224,33.856));
#60883=CARTESIAN_POINT('',(-13.4871572875254,1.224,31.1888427124746));
#60884=CARTESIAN_POINT('',(16.1543145750508,1.224,33.856));
#60885=CARTESIAN_POINT('',(8.16,1.224,33.856));
#60886=CARTESIAN_POINT('',(18.368,1.224,36.0696854249492));
#60887=CARTESIAN_POINT('',(14.7111572875254,1.224,32.4128427124746));
#60888=CARTESIAN_POINT('',(18.368,1.224,42.636));
#60889=CARTESIAN_POINT('',(-15.904,1.224,41.208));
#60890=CARTESIAN_POINT('',(-14.8512,1.224,41.208));
#60891=CARTESIAN_POINT('',(-7.752,1.224,41.208));
#60892=CARTESIAN_POINT('',(-14.8512,1.224,42.432));
#60893=CARTESIAN_POINT('',(-14.8512,1.224,41.004));
#60894=CARTESIAN_POINT('',(-13.7088,1.224,42.432));
#60895=CARTESIAN_POINT('',(-6.8544,1.224,42.432));
#60896=CARTESIAN_POINT('',(-13.7088,1.224,41.208));
#60897=CARTESIAN_POINT('',(-13.7088,1.224,38.2296));
#60898=CARTESIAN_POINT('',(-12.656,1.224,41.208));
#60899=CARTESIAN_POINT('',(-7.752,1.224,41.208));
#60900=CARTESIAN_POINT('',(-12.656,1.224,35.504));
#60901=CARTESIAN_POINT('',(-12.656,1.224,40.392));
#60902=CARTESIAN_POINT('',(-15.904,1.224,35.504));
#60903=CARTESIAN_POINT('',(-6.528,1.224,35.504));
#60904=CARTESIAN_POINT('',(-15.904,1.224,37.74));
#60905=CARTESIAN_POINT('',(12.656,1.224,41.208));
#60906=CARTESIAN_POINT('',(13.7088,1.224,41.208));
#60907=CARTESIAN_POINT('',(6.528,1.224,41.208));
#60908=CARTESIAN_POINT('',(13.7088,1.224,42.432));
#60909=CARTESIAN_POINT('',(13.7088,1.224,41.004));
#60910=CARTESIAN_POINT('',(14.8512,1.224,42.432));
#60911=CARTESIAN_POINT('',(7.4256,1.224,42.432));
#60912=CARTESIAN_POINT('',(14.8512,1.224,41.208));
#60913=CARTESIAN_POINT('',(14.8512,1.224,38.2296));
#60914=CARTESIAN_POINT('',(15.904,1.224,41.208));
#60915=CARTESIAN_POINT('',(6.528,1.224,41.208));
#60916=CARTESIAN_POINT('',(15.904,1.224,35.504));
#60917=CARTESIAN_POINT('',(15.904,1.224,40.392));
#60918=CARTESIAN_POINT('',(12.656,1.224,35.504));
#60919=CARTESIAN_POINT('',(7.752,1.224,35.504));
#60920=CARTESIAN_POINT('',(12.656,1.224,37.74));
#60921=CARTESIAN_POINT('',(-6.528,1.224,40.732));
#60922=CARTESIAN_POINT('Origin',(-6.528,1.224,42.432));
#60923=CARTESIAN_POINT('Origin',(8.16,1.624,33.856));
#60924=CARTESIAN_POINT('Origin',(-16.1543145750508,1.624,33.856));
#60925=CARTESIAN_POINT('Origin',(16.1543145750508,1.624,33.856));
#60926=CARTESIAN_POINT('Origin',(-13.4871572875254,1.624,31.1888427124746));
#60927=CARTESIAN_POINT('Origin',(18.368,1.624,42.636));
#60928=CARTESIAN_POINT('Origin',(18.368,1.624,36.0696854249492));
#60929=CARTESIAN_POINT('Origin',(14.7111572875254,1.624,32.4128427124746));
#60930=CARTESIAN_POINT('Origin',(-6.528,1.624,42.432));
#60931=CARTESIAN_POINT('',(-6.528,1.624,41.132));
#60932=CARTESIAN_POINT('Origin',(-6.528,1.624,40.732));
#60933=CARTESIAN_POINT('',(-7.828,1.624,42.432));
#60934=CARTESIAN_POINT('Origin',(-6.528,1.624,42.432));
#60935=CARTESIAN_POINT('Origin',(-6.528,1.624,42.432));
#60936=CARTESIAN_POINT('Origin',(-6.528,1.224,42.432));
#60937=CARTESIAN_POINT('',(-7.828,2.048,42.432));
#60938=CARTESIAN_POINT('',(-7.828,1.224,42.432));
#60939=CARTESIAN_POINT('',(-6.528,2.048,43.732));
#60940=CARTESIAN_POINT('Origin',(-6.528,2.048,42.432));
#60941=CARTESIAN_POINT('Origin',(-6.528,2.048,42.432));
#60942=CARTESIAN_POINT('Origin',(-6.528,2.048,42.432));
#60943=CARTESIAN_POINT('Origin',(-6.528,2.048,44.132));
#60944=CARTESIAN_POINT('Origin',(12.656,2.048,37.74));
#60945=CARTESIAN_POINT('',(13.056,2.048,41.208));
#60946=CARTESIAN_POINT('Origin',(12.656,2.048,41.608));
#60947=CARTESIAN_POINT('',(13.056,2.048,35.904));
#60948=CARTESIAN_POINT('',(13.056,2.048,37.74));
#60949=CARTESIAN_POINT('Origin',(12.656,2.048,35.504));
#60950=CARTESIAN_POINT('Origin',(6.528,2.048,41.608));
#60951=CARTESIAN_POINT('',(15.504,2.048,41.208));
#60952=CARTESIAN_POINT('',(6.528,2.048,41.208));
#60953=CARTESIAN_POINT('Origin',(15.904,2.048,41.608));
#60954=CARTESIAN_POINT('Origin',(7.752,2.048,35.504));
#60955=CARTESIAN_POINT('',(15.504,2.048,35.904));
#60956=CARTESIAN_POINT('',(7.752,2.048,35.904));
#60957=CARTESIAN_POINT('Origin',(15.904,2.048,35.504));
#60958=CARTESIAN_POINT('Origin',(15.904,2.048,40.392));
#60959=CARTESIAN_POINT('',(15.504,2.048,40.392));
#60960=CARTESIAN_POINT('Origin',(15.504,1.224,35.904));
#60961=CARTESIAN_POINT('',(13.056,1.624,35.904));
#60962=CARTESIAN_POINT('',(13.056,1.224,35.904));
#60963=CARTESIAN_POINT('',(15.504,1.624,35.904));
#60964=CARTESIAN_POINT('',(7.752,1.624,35.904));
#60965=CARTESIAN_POINT('',(15.504,1.224,35.904));
#60966=CARTESIAN_POINT('Origin',(13.056,1.224,35.904));
#60967=CARTESIAN_POINT('',(13.056,1.624,41.208));
#60968=CARTESIAN_POINT('',(13.056,1.224,41.208));
#60969=CARTESIAN_POINT('',(13.056,1.624,37.74));
#60970=CARTESIAN_POINT('Origin',(12.656,1.624,37.74));
#60971=CARTESIAN_POINT('Origin',(12.656,1.624,41.208));
#60972=CARTESIAN_POINT('Origin',(12.656,1.624,35.504));
#60973=CARTESIAN_POINT('Origin',(7.752,1.624,35.504));
#60974=CARTESIAN_POINT('Origin',(15.904,1.624,35.504));
#60975=CARTESIAN_POINT('Origin',(15.904,1.624,40.392));
#60976=CARTESIAN_POINT('',(15.504,1.624,41.208));
#60977=CARTESIAN_POINT('Origin',(15.904,1.624,41.208));
#60978=CARTESIAN_POINT('',(15.504,1.624,40.392));
#60979=CARTESIAN_POINT('Origin',(15.504,1.224,41.208));
#60980=CARTESIAN_POINT('',(15.504,1.224,41.208));
#60981=CARTESIAN_POINT('Origin',(-15.904,2.048,37.74));
#60982=CARTESIAN_POINT('',(-15.504,2.048,41.208));
#60983=CARTESIAN_POINT('Origin',(-15.904,2.048,41.608));
#60984=CARTESIAN_POINT('',(-15.504,2.048,35.904));
#60985=CARTESIAN_POINT('',(-15.504,2.048,37.74));
#60986=CARTESIAN_POINT('Origin',(-15.904,2.048,35.504));
#60987=CARTESIAN_POINT('Origin',(-7.752,2.048,41.608));
#60988=CARTESIAN_POINT('',(-13.056,2.048,41.208));
#60989=CARTESIAN_POINT('',(-7.752,2.048,41.208));
#60990=CARTESIAN_POINT('Origin',(-12.656,2.048,41.608));
#60991=CARTESIAN_POINT('Origin',(-6.528,2.048,35.504));
#60992=CARTESIAN_POINT('',(-13.056,2.048,35.904));
#60993=CARTESIAN_POINT('',(-6.528,2.048,35.904));
#60994=CARTESIAN_POINT('Origin',(-12.656,2.048,35.504));
#60995=CARTESIAN_POINT('Origin',(-12.656,2.048,40.392));
#60996=CARTESIAN_POINT('',(-13.056,2.048,40.392));
#60997=CARTESIAN_POINT('Origin',(-13.056,1.224,35.904));
#60998=CARTESIAN_POINT('',(-15.504,1.624,35.904));
#60999=CARTESIAN_POINT('',(-15.504,1.224,35.904));
#61000=CARTESIAN_POINT('',(-13.056,1.624,35.904));
#61001=CARTESIAN_POINT('',(-6.528,1.624,35.904));
#61002=CARTESIAN_POINT('',(-13.056,1.224,35.904));
#61003=CARTESIAN_POINT('Origin',(-15.504,1.224,35.904));
#61004=CARTESIAN_POINT('',(-15.504,1.624,41.208));
#61005=CARTESIAN_POINT('',(-15.504,1.224,41.208));
#61006=CARTESIAN_POINT('',(-15.504,1.624,37.74));
#61007=CARTESIAN_POINT('Origin',(-15.904,1.624,37.74));
#61008=CARTESIAN_POINT('Origin',(-15.904,1.624,41.208));
#61009=CARTESIAN_POINT('Origin',(-15.904,1.624,35.504));
#61010=CARTESIAN_POINT('Origin',(-6.528,1.624,35.504));
#61011=CARTESIAN_POINT('Origin',(-12.656,1.624,35.504));
#61012=CARTESIAN_POINT('Origin',(-12.656,1.624,40.392));
#61013=CARTESIAN_POINT('',(-13.056,1.624,41.208));
#61014=CARTESIAN_POINT('Origin',(-12.656,1.624,41.208));
#61015=CARTESIAN_POINT('',(-13.056,1.624,40.392));
#61016=CARTESIAN_POINT('Origin',(-13.056,1.224,41.208));
#61017=CARTESIAN_POINT('',(-13.056,1.224,41.208));
#61018=CARTESIAN_POINT('Origin',(14.1088,0.8896,41.0448));
#61019=CARTESIAN_POINT('',(13.7101470682411,0.8568,36.8832));
#61020=CARTESIAN_POINT('',(14.1088,0.4896,36.8832));
#61021=CARTESIAN_POINT('Origin',(14.1088,0.8896,36.8832));
#61022=CARTESIAN_POINT('',(14.1088,0.4896,42.432));
#61023=CARTESIAN_POINT('',(14.1088,0.4896,41.0448));
#61024=CARTESIAN_POINT('',(13.7088,0.8896,42.432));
#61025=CARTESIAN_POINT('Origin',(14.1088,0.8896,42.432));
#61026=CARTESIAN_POINT('',(13.7088,0.8896,41.208));
#61027=CARTESIAN_POINT('',(13.7088,0.8896,41.0448));
#61028=CARTESIAN_POINT('',(13.7101470682411,0.8568,41.208));
#61029=CARTESIAN_POINT('Origin',(14.1088,0.8896,41.208));
#61030=CARTESIAN_POINT('',(13.7101470682411,0.8568,41.0448));
#61031=CARTESIAN_POINT('Origin',(14.1088,0.824,41.0448));
#61032=CARTESIAN_POINT('',(14.1088,1.224,41.208));
#61033=CARTESIAN_POINT('Origin',(14.1088,0.824,41.208));
#61034=CARTESIAN_POINT('',(14.1088,1.224,36.8832));
#61035=CARTESIAN_POINT('',(14.1088,1.224,41.0448));
#61036=CARTESIAN_POINT('Origin',(14.1088,0.824,36.8832));
#61037=CARTESIAN_POINT('Origin',(13.056,1.224,41.208));
#61038=CARTESIAN_POINT('',(14.8512,0.8896,41.208));
#61039=CARTESIAN_POINT('',(14.8512,1.224,41.208));
#61040=CARTESIAN_POINT('',(14.8498529317589,0.8568,41.208));
#61041=CARTESIAN_POINT('Origin',(14.4512,0.8896,41.208));
#61042=CARTESIAN_POINT('',(14.4512,1.224,41.208));
#61043=CARTESIAN_POINT('Origin',(14.4512,0.824,41.208));
#61044=CARTESIAN_POINT('',(6.528,1.224,41.208));
#61045=CARTESIAN_POINT('',(13.7088,1.224,41.208));
#61046=CARTESIAN_POINT('Origin',(13.7088,1.224,42.432));
#61047=CARTESIAN_POINT('',(13.7088,1.224,42.432));
#61048=CARTESIAN_POINT('Origin',(13.7088,1.224,36.8832));
#61049=CARTESIAN_POINT('',(14.4512,1.224,36.8832));
#61050=CARTESIAN_POINT('',(13.7088,1.224,36.8832));
#61051=CARTESIAN_POINT('',(14.8498529317589,0.8568,36.8832));
#61052=CARTESIAN_POINT('Origin',(14.4512,0.824,36.8832));
#61053=CARTESIAN_POINT('',(14.4512,0.4896,36.8832));
#61054=CARTESIAN_POINT('Origin',(14.4512,0.8896,36.8832));
#61055=CARTESIAN_POINT('',(13.7088,0.4896,36.8832));
#61056=CARTESIAN_POINT('Origin',(14.4512,0.8896,38.2704));
#61057=CARTESIAN_POINT('',(14.8512,0.8896,42.432));
#61058=CARTESIAN_POINT('',(14.4512,0.4896,42.432));
#61059=CARTESIAN_POINT('Origin',(14.4512,0.8896,42.432));
#61060=CARTESIAN_POINT('',(14.4512,0.4896,38.2704));
#61061=CARTESIAN_POINT('',(14.8498529317589,0.8568,38.2704));
#61062=CARTESIAN_POINT('',(14.8512,0.8896,38.2704));
#61063=CARTESIAN_POINT('Origin',(14.28,0.4896,39.6576));
#61064=CARTESIAN_POINT('',(14.8512,0.4896,42.432));
#61065=CARTESIAN_POINT('Origin',(14.8512,1.224,42.432));
#61066=CARTESIAN_POINT('',(14.8512,1.224,42.432));
#61067=CARTESIAN_POINT('Origin',(14.8512,1.224,36.8832));
#61068=CARTESIAN_POINT('Origin',(14.4512,0.824,38.2704));
#61069=CARTESIAN_POINT('',(14.4512,1.224,38.2704));
#61070=CARTESIAN_POINT('Origin',(-14.4512,0.8896,41.0448));
#61071=CARTESIAN_POINT('',(-14.8498529317589,0.8568,36.8832));
#61072=CARTESIAN_POINT('',(-14.4512,0.4896,36.8832));
#61073=CARTESIAN_POINT('Origin',(-14.4512,0.8896,36.8832));
#61074=CARTESIAN_POINT('',(-14.4512,0.4896,42.432));
#61075=CARTESIAN_POINT('',(-14.4512,0.4896,41.0448));
#61076=CARTESIAN_POINT('',(-14.8512,0.8896,42.432));
#61077=CARTESIAN_POINT('Origin',(-14.4512,0.8896,42.432));
#61078=CARTESIAN_POINT('',(-14.8512,0.8896,41.208));
#61079=CARTESIAN_POINT('',(-14.8512,0.8896,41.0448));
#61080=CARTESIAN_POINT('',(-14.8498529317589,0.8568,41.208));
#61081=CARTESIAN_POINT('Origin',(-14.4512,0.8896,41.208));
#61082=CARTESIAN_POINT('',(-14.8498529317589,0.8568,41.0448));
#61083=CARTESIAN_POINT('Origin',(-14.4512,0.824,41.0448));
#61084=CARTESIAN_POINT('',(-14.4512,1.224,41.208));
#61085=CARTESIAN_POINT('Origin',(-14.4512,0.824,41.208));
#61086=CARTESIAN_POINT('',(-14.4512,1.224,36.8832));
#61087=CARTESIAN_POINT('',(-14.4512,1.224,41.0448));
#61088=CARTESIAN_POINT('Origin',(-14.4512,0.824,36.8832));
#61089=CARTESIAN_POINT('Origin',(-15.504,1.224,41.208));
#61090=CARTESIAN_POINT('',(-13.7088,0.8896,41.208));
#61091=CARTESIAN_POINT('',(-13.7088,1.224,41.208));
#61092=CARTESIAN_POINT('',(-13.7101470682411,0.8568,41.208));
#61093=CARTESIAN_POINT('Origin',(-14.1088,0.8896,41.208));
#61094=CARTESIAN_POINT('',(-14.1088,1.224,41.208));
#61095=CARTESIAN_POINT('Origin',(-14.1088,0.824,41.208));
#61096=CARTESIAN_POINT('',(-7.752,1.224,41.208));
#61097=CARTESIAN_POINT('',(-14.8512,1.224,41.208));
#61098=CARTESIAN_POINT('Origin',(-14.8512,1.224,42.432));
#61099=CARTESIAN_POINT('',(-14.8512,1.224,42.432));
#61100=CARTESIAN_POINT('Origin',(-14.8512,1.224,36.8832));
#61101=CARTESIAN_POINT('',(-14.1088,1.224,36.8832));
#61102=CARTESIAN_POINT('',(-14.8512,1.224,36.8832));
#61103=CARTESIAN_POINT('',(-13.7101470682411,0.8568,36.8832));
#61104=CARTESIAN_POINT('Origin',(-14.1088,0.824,36.8832));
#61105=CARTESIAN_POINT('',(-14.1088,0.4896,36.8832));
#61106=CARTESIAN_POINT('Origin',(-14.1088,0.8896,36.8832));
#61107=CARTESIAN_POINT('',(-14.8512,0.4896,36.8832));
#61108=CARTESIAN_POINT('Origin',(-14.1088,0.8896,38.2704));
#61109=CARTESIAN_POINT('',(-13.7088,0.8896,42.432));
#61110=CARTESIAN_POINT('',(-14.1088,0.4896,42.432));
#61111=CARTESIAN_POINT('Origin',(-14.1088,0.8896,42.432));
#61112=CARTESIAN_POINT('',(-14.1088,0.4896,38.2704));
#61113=CARTESIAN_POINT('',(-13.7101470682411,0.8568,38.2704));
#61114=CARTESIAN_POINT('',(-13.7088,0.8896,38.2704));
#61115=CARTESIAN_POINT('Origin',(-14.28,0.4896,39.6576));
#61116=CARTESIAN_POINT('',(-13.7088,0.4896,42.432));
#61117=CARTESIAN_POINT('Origin',(-13.7088,1.224,42.432));
#61118=CARTESIAN_POINT('',(-13.7088,1.224,42.432));
#61119=CARTESIAN_POINT('Origin',(-13.7088,1.224,36.8832));
#61120=CARTESIAN_POINT('Origin',(-14.1088,0.824,38.2704));
#61121=CARTESIAN_POINT('',(-14.1088,1.224,38.2704));
#61122=CARTESIAN_POINT('Origin',(-14.28,1.224,39.6576));
#61123=CARTESIAN_POINT('Origin',(14.28,1.224,39.6576));
#61124=CARTESIAN_POINT('Origin',(-17.544,8.976,41.616));
#61125=CARTESIAN_POINT('Origin',(-17.544,21.216,32.64));
#61126=CARTESIAN_POINT('Origin',(17.544,8.976,38.76));
#99995=UNCERTAINTY_MEASURE_WITH_UNIT(LENGTH_MEASURE(0.01),#100032,
'DISTANCE_ACCURACY_VALUE',
'Maximum model space distance between geometric entities at asserted c
onnectivities');
#100011=UNCERTAINTY_MEASURE_WITH_UNIT(LENGTH_MEASURE(0.01),#100032,
'DISTANCE_ACCURACY_VALUE',
'Maximum model space distance between geometric entities at asserted c
onnectivities');
#100015=(
GEOMETRIC_REPRESENTATION_CONTEXT(3)
GLOBAL_UNCERTAINTY_ASSIGNED_CONTEXT((#99995))
GLOBAL_UNIT_ASSIGNED_CONTEXT((#100032,#100034,#100035))
REPRESENTATION_CONTEXT('','3D')
);
#100031=(
GEOMETRIC_REPRESENTATION_CONTEXT(3)
GLOBAL_UNCERTAINTY_ASSIGNED_CONTEXT((#100011))
GLOBAL_UNIT_ASSIGNED_CONTEXT((#100032,#100034,#100035))
REPRESENTATION_CONTEXT('','3D')
);
#100032=(
LENGTH_UNIT()
NAMED_UNIT(*)
SI_UNIT(.MILLI.,.METRE.)
);
#100034=(
NAMED_UNIT(*)
PLANE_ANGLE_UNIT()
SI_UNIT($,.RADIAN.)
);
#100035=(
NAMED_UNIT(*)
SI_UNIT($,.STERADIAN.)
SOLID_ANGLE_UNIT()
);
#100039=SHAPE_DEFINITION_REPRESENTATION(#100058,#100103);
#100058=PRODUCT_DEFINITION_SHAPE('',$,#100123);
#100103=SHAPE_REPRESENTATION('',(#20892),#100015);
#100119=PRODUCT_DEFINITION_CONTEXT('part definition',#100178,'design');
#100123=PRODUCT_DEFINITION('2026-10-12-11-54-54-063',
'03_Coupling_Bracket_U-Channel',#100142,#100119);
#100142=PRODUCT_DEFINITION_FORMATION('',$,#100183);
#100178=APPLICATION_CONTEXT(
'Core Data for Automotive Mechanical Design Process');
#100179=PRODUCT_CONTEXT('part definition',#100178,'mechanical');
#100183=PRODUCT('2026-10-12-11-54-54-063',
'03_Coupling_Bracket_U-Channel',$,(#100179));
#100201=PRESENTATION_STYLE_ASSIGNMENT((#100207));
#100207=SURFACE_STYLE_USAGE(.BOTH.,#100213);
#100213=SURFACE_SIDE_STYLE('',(#100219));
#100219=SURFACE_STYLE_FILL_AREA(#100225);
#100225=FILL_AREA_STYLE('Opaque(20,51,87)',(#100231));
#100231=FILL_AREA_STYLE_COLOUR('Opaque(20,51,87)',#100237);
#100237=COLOUR_RGB('Opaque(20,51,87)',0.0784313725490196,0.2,0.341176470588235);
ENDSEC;
END-ISO-10303-21;
